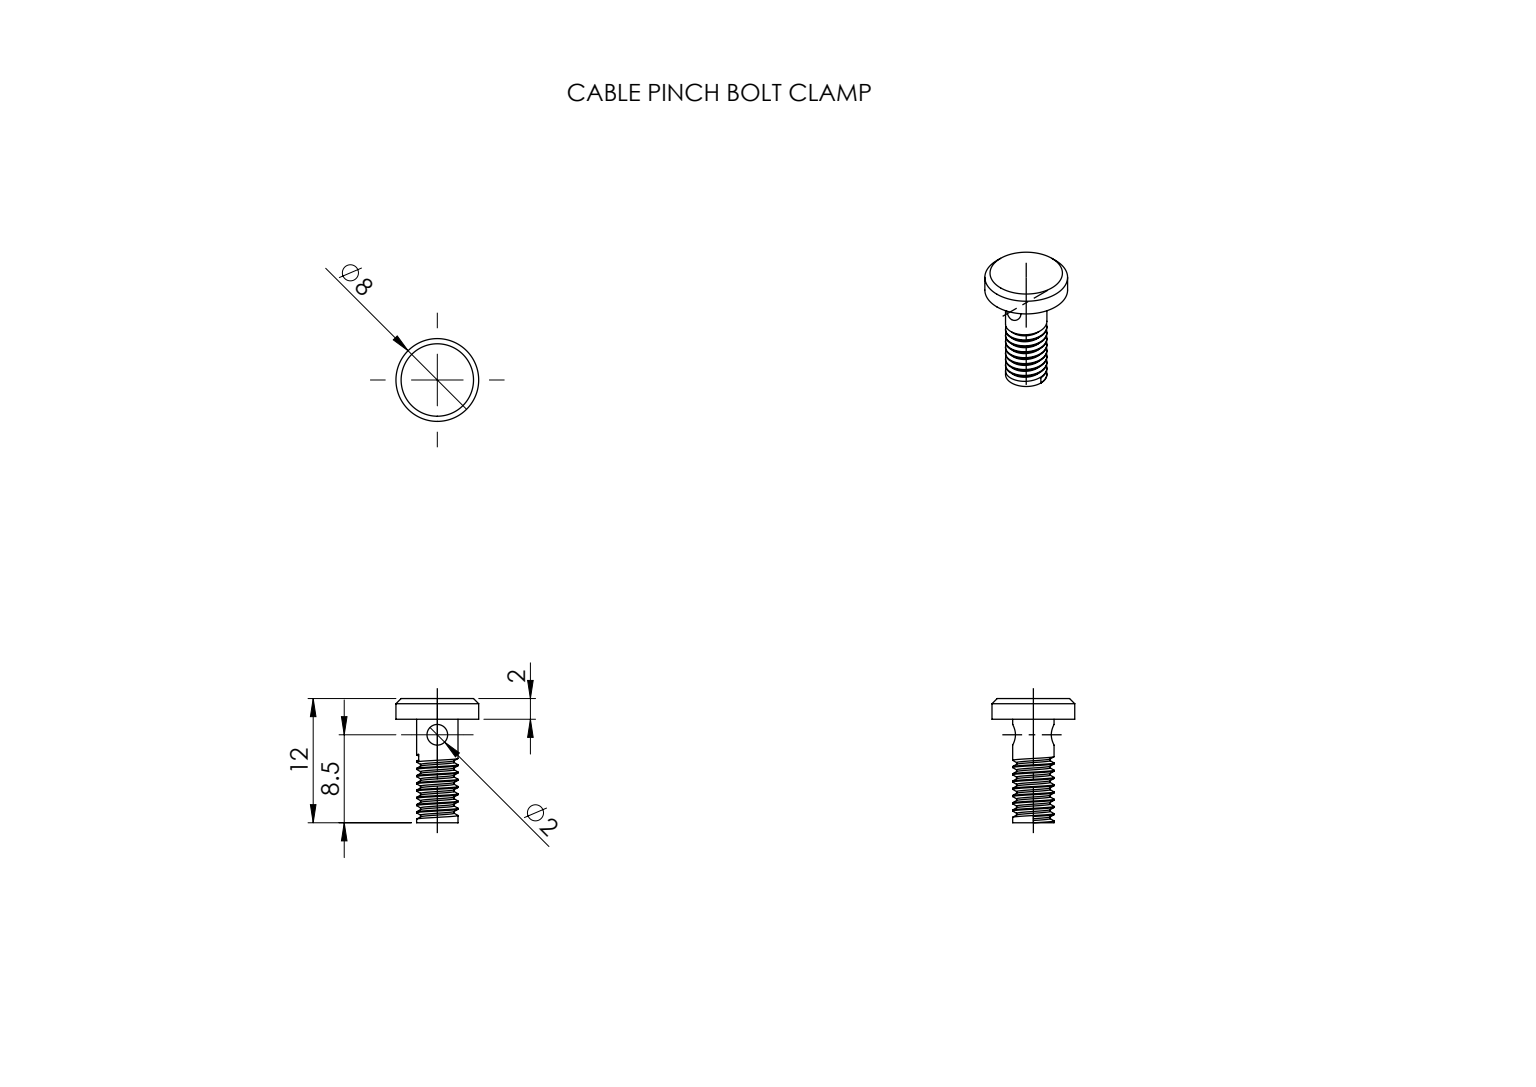
ISO-10303-21;
HEADER;
FILE_DESCRIPTION (('STEP AP214'),
    '1' );
FILE_NAME ('Cable Pinch Bolt Clamp.step',
    '2026-10-08T05:45:04',
    ( '' ),
    ( '' ),
    'SwSTEP 2.0',
    'SolidWorks 2026',
    '' );
FILE_SCHEMA (( 'AUTOMOTIVE_DESIGN' ));
ENDSEC;

DATA;
#6=CARTESIAN_POINT ( 'NONE',  ( -25.98076211353311393, 52.34374999904395054, -3.128098921329806714 ) ) ;
#9=( BOUNDED_CURVE ( )  B_SPLINE_CURVE ( 2, ( #10910, #4195, #7581, #6742, #4979, #7521, #70, #5149, #6620 ),
 .UNSPECIFIED., .F., .F. ) 
 B_SPLINE_CURVE_WITH_KNOTS ( ( 3, 2, 2, 2, 3 ),
 ( 0.6944444444444445308, 0.7037037037037037202, 0.7222222222222222099, 0.7407407407407406996, 0.7500000000000000000 ),
 .UNSPECIFIED. ) 
 CURVE ( )  GEOMETRIC_REPRESENTATION_ITEM ( )  RATIONAL_B_SPLINE_CURVE ( ( 0.9330127018922194093, 0.9330127018922197424, 1.000000000000000000, 0.8660254037844387076, 1.000000000000000000, 0.8660254037844387076, 1.000000000000000000, 0.9330127018922194093, 0.9330127018922194093 ) ) 
 REPRESENTATION_ITEM ( '' )  );
#14=DIRECTION ( 'NONE',  ( 0.000000000000000000, 0.000000000000000000, 1.000000000000000000 ) ) ;
#22=CARTESIAN_POINT ( 'NONE',  ( -24.35964822603314417, 53.91874999904395338, -5.000000000000103029 ) ) ;
#30=CARTESIAN_POINT ( 'NONE',  ( -25.98076211353311038, 60.99999999999985789, -0.9999999999995021760 ) ) ;
#31=CARTESIAN_POINT ( 'NONE',  ( -24.35964822603314772, 52.63541666571061484, -4.064049460664953983 ) ) ;
#32=CARTESIAN_POINT ( 'NONE',  ( -24.35964822603314772, 55.26041666571061484, -4.064049460664953983 ) ) ;
#35=CARTESIAN_POINT ( 'NONE',  ( -26.98076211353309972, 53.23333333333319217, -6.732050807568954909 ) ) ;
#47=CARTESIAN_POINT ( 'NONE',  ( -25.17020516978313083, 50.01041666571061484, -6.403925809002825709 ) ) ;
#52=CARTESIAN_POINT ( 'NONE',  ( -24.35964822603314417, 49.89374999904394770, -5.000000000000103029 ) ) ;
#54=ORIENTED_EDGE ( 'NONE', *, *, #4990, .T. ) ;
#62=CARTESIAN_POINT ( 'NONE',  ( -26.79131905728310059, 52.28541666571062052, -3.596074190997381237 ) ) ;
#65=CARTESIAN_POINT ( 'NONE',  ( -26.85195975805010704, 58.50831236826149251, -6.801198016534330648 ) ) ;
#67=ORIENTED_EDGE ( 'NONE', *, *, #8603, .T. ) ;
#68=AXIS2_PLACEMENT_3D ( 'NONE', #5659, #5549, #6578 ) ;
#70=CARTESIAN_POINT ( 'NONE',  ( -26.98076211353309972, 54.77916666475469754, -3.267949192431252037 ) ) ;
#74=DIRECTION ( 'NONE',  ( 1.000000000000000000, 0.000000000000000000, 0.000000000000000000 ) ) ;
#77=CARTESIAN_POINT ( 'NONE',  ( -25.98076211353311393, 55.49374999904395622, -6.871901078670400231 ) ) ;
#85=CARTESIAN_POINT ( 'NONE',  ( -25.98076211353311393, 54.22499999999985931, -3.000000000000132339 ) ) ;
#88=CARTESIAN_POINT ( 'NONE',  ( -24.35964822603314417, 52.69374999904394485, -5.000000000000103029 ) ) ;
#93=CARTESIAN_POINT ( 'NONE',  ( -27.98076211353308551, 54.69166666666652787, -6.154700538379338504 ) ) ;
#101=VERTEX_POINT ( 'NONE', #7634 ) ;
#106=CARTESIAN_POINT ( 'NONE',  ( -25.17020516978313083, 50.71041666571061057, -6.403925809002825709 ) ) ;
#111=CARTESIAN_POINT ( 'NONE',  ( -27.60187600103308014, 50.88541666571062194, -5.935950539335252074 ) ) ;
#114=CARTESIAN_POINT ( 'NONE',  ( -25.84804642293430277, 59.00000000000105871, -3.000000000000019984 ) ) ;
#123=CARTESIAN_POINT ( 'NONE',  ( -26.79131905728310059, 50.65208333237728766, -6.403925809002825709 ) ) ;
#128=ORIENTED_EDGE ( 'NONE', *, *, #2197, .F. ) ;
#130=ORIENTED_EDGE ( 'NONE', *, *, #7314, .T. ) ;
#133=DIRECTION ( 'NONE',  ( 0.000000000000000000, 1.000000000000000000, 0.000000000000000000 ) ) ;
#137=CARTESIAN_POINT ( 'NONE',  ( -26.98076211353309972, 52.76666666666653072, -3.267949192431252037 ) ) ;
#139=CARTESIAN_POINT ( 'NONE',  ( -24.35964822603314772, 54.56041666571061910, -4.064049460664953983 ) ) ;
#149=CARTESIAN_POINT ( 'NONE',  ( -24.35964822603314417, 55.49374999904394912, -5.000000000000103029 ) ) ;
#154=CARTESIAN_POINT ( 'NONE',  ( -23.98076211353314235, 54.39999999999986358, -5.000000000000103029 ) ) ;
#160=PRODUCT_CONTEXT ( 'NONE', #1750, 'mechanical' ) ;
#163=CARTESIAN_POINT ( 'NONE',  ( -23.98076211353314235, 54.34166666666652645, -3.845299461620867554 ) ) ;
#168=CARTESIAN_POINT ( 'NONE',  ( -26.79131905728310059, 53.86041666571061626, -3.596074190997381237 ) ) ;
#178=DIRECTION ( 'NONE',  ( -2.775557561562891351E-17, -1.000000000000000000, 8.326672684688671588E-17 ) ) ;
#179=CARTESIAN_POINT ( 'NONE',  ( -26.79131905728310059, 52.05208333237728624, -6.403925809002825709 ) ) ;
#186=CARTESIAN_POINT ( 'NONE',  ( -25.98076211353311393, 49.49999999999986500, -5.000000000000103029 ) ) ;
#187=FACE_OUTER_BOUND ( 'NONE', #10441, .T. ) ;
#189=CARTESIAN_POINT ( 'NONE',  ( -25.17020516978313083, 55.43541666571061910, -6.403925809002825709 ) ) ;
#190=CYLINDRICAL_SURFACE ( 'NONE', #9308, 1.999999999999971356 ) ;
#199=CARTESIAN_POINT ( 'NONE',  ( -26.98076211353408382, 57.99999999999985789, -6.732050807568389139 ) ) ;
#200=CARTESIAN_POINT ( 'NONE',  ( -23.98076211353314235, 55.15833333333319644, -6.154700538379337615 ) ) ;
#214=CARTESIAN_POINT ( 'NONE',  ( -25.98076211353311393, 54.26874999904394059, -6.871901078670400231 ) ) ;
#215=LINE ( 'NONE', #1106, #6427 ) ;
#229=CARTESIAN_POINT ( 'NONE',  ( -26.79131905728310059, 51.58541666571061768, -3.596074190997381237 ) ) ;
#232=FACE_OUTER_BOUND ( 'NONE', #6046, .T. ) ;
#239=CARTESIAN_POINT ( 'NONE',  ( -27.44132740410865523, 55.89336612041927310, -4.296608737464627126 ) ) ;
#243=SURFACE_SIDE_STYLE ('',( #1130 ) ) ;
#251=CARTESIAN_POINT ( 'NONE',  ( -26.98076211353408382, 57.86742347890963600, -6.732050807568390027 ) ) ;
#256=CARTESIAN_POINT ( 'NONE',  ( -26.98076211353309972, 55.33333333333320070, -6.732050807568954909 ) ) ;
#260=CIRCLE ( 'NONE', #5589, 4.000000000000600409 ) ;
#261=EDGE_LOOP ( 'NONE', ( #3712, #6126, #2093, #9383 ) ) ;
#273=CARTESIAN_POINT ( 'NONE',  ( -24.35964822603314772, 51.23541666571061626, -4.064049460664953983 ) ) ;
#276=VERTEX_POINT ( 'NONE', #6124 ) ;
#287=CARTESIAN_POINT ( 'NONE',  ( -27.60187600103308370, 55.66874999904394627, -5.000000000000103029 ) ) ;
#288=FACE_OUTER_BOUND ( 'NONE', #1831, .T. ) ;
#293=EDGE_CURVE ( 'NONE', #9873, #5764, #10428, .T. ) ;
#294=CARTESIAN_POINT ( 'NONE',  ( -27.78268512908116961, 55.49961679590672503, -4.132201955500060642 ) ) ;
#297=LINE ( 'NONE', #1976, #5079 ) ;
#308=AXIS2_PLACEMENT_3D ( 'NONE', #6956, #4296, #9565 ) ;
#311=CARTESIAN_POINT ( 'NONE',  ( -24.98076211353313170, 54.89583333142136468, -3.267949192431250705 ) ) ;
#313=CARTESIAN_POINT ( 'NONE',  ( -25.98076211353311393, 54.26874999904394059, -6.871901078670400231 ) ) ;
#315=AXIS2_PLACEMENT_3D ( 'NONE', #3172, #7503, #4003 ) ;
#325=CARTESIAN_POINT ( 'NONE',  ( -25.98076211353310683, 49.89374999904395480, -6.871901078670399343 ) ) ;
#328=ORIENTED_EDGE ( 'NONE', *, *, #9673, .F. ) ;
#329=CARTESIAN_POINT ( 'NONE',  ( -27.60187600103308370, 53.04374999904394627, -5.000000000000103029 ) ) ;
#339=CARTESIAN_POINT ( 'NONE',  ( -25.98076211353311393, 54.44374999904394485, -3.128098921329806714 ) ) ;
#341=CARTESIAN_POINT ( 'NONE',  ( -25.44486372867087454, 53.05623925897106830, -7.000000000000073719 ) ) ;
#357=CARTESIAN_POINT ( 'NONE',  ( -26.85338401696505883, 57.49468158336109269, -6.800474515642543238 ) ) ;
#362=CARTESIAN_POINT ( 'NONE',  ( -26.79131905728310059, 52.92708333237727913, -6.403925809002825709 ) ) ;
#367=CARTESIAN_POINT ( 'NONE',  ( -25.98076211353310683, 54.92499999999986926, -3.000000000000132339 ) ) ;
#378=CARTESIAN_POINT ( 'NONE',  ( -24.35964822603314772, 54.73541666571060915, -4.064049460664953983 ) ) ;
#388=CARTESIAN_POINT ( 'NONE',  ( -27.98076211353308551, 49.84999999999986642, -5.000000000000103029 ) ) ;
#399=CARTESIAN_POINT ( 'NONE',  ( -25.98076211353311393, 55.88749999808803182, -7.000000000000072831 ) ) ;
#404=ORIENTED_EDGE ( 'NONE', *, *, #1797, .F. ) ;
#409=EDGE_CURVE ( 'NONE', #4738, #10440, #8087, .T. ) ;
#413=CARTESIAN_POINT ( 'NONE',  ( -24.35964822603314417, 52.69374999904394485, -5.000000000000103029 ) ) ;
#433=VERTEX_POINT ( 'NONE', #9014 ) ;
#453=CARTESIAN_POINT ( 'NONE',  ( -25.44486372867087454, 52.44373926088289295, -7.000000000000073719 ) ) ;
#455=CARTESIAN_POINT ( 'NONE',  ( -25.47388223254686324, 57.12817616725342162, -6.938581062208108108 ) ) ;
#467=CARTESIAN_POINT ( 'NONE',  ( -25.44486372867087809, 52.35623925897106545, -7.000000000000075495 ) ) ;
#469=CARTESIAN_POINT ( 'NONE',  ( -23.98076211353314235, 51.54166666666652219, -3.845299461620867554 ) ) ;
#470=CARTESIAN_POINT ( 'NONE',  ( -24.35964822603314417, 53.39374999904394770, -5.000000000000103029 ) ) ;
#474=ORIENTED_EDGE ( 'NONE', *, *, #7144, .T. ) ;
#482=CARTESIAN_POINT ( 'NONE',  ( -25.98076211353310683, 51.29374999904394627, -6.871901078670399343 ) ) ;
#483=AXIS2_PLACEMENT_3D ( 'NONE', #5841, #2237, #5628 ) ;
#491=VERTEX_POINT ( 'NONE', #504 ) ;
#503=CARTESIAN_POINT ( 'NONE',  ( -27.98076211353308551, 51.80416666475470322, -6.154700538379338504 ) ) ;
#504=CARTESIAN_POINT ( 'NONE',  ( -25.98076211353311393, 51.77499999999986358, -7.000000000000072831 ) ) ;
#507=EDGE_LOOP ( 'NONE', ( #5439, #6866, #1397, #7624 ) ) ;
#509=LINE ( 'NONE', #4853, #3476 ) ;
#511=CARTESIAN_POINT ( 'NONE',  ( -27.98076211353308551, 52.50416666475469896, -6.154700538379338504 ) ) ;
#522=CARTESIAN_POINT ( 'NONE',  ( -25.98076211353311393, 51.07499999999986784, -7.000000000000073719 ) ) ;
#523=CARTESIAN_POINT ( 'NONE',  ( -24.35964822603314772, 54.03541666571061342, -4.064049460664953983 ) ) ;
#525=CARTESIAN_POINT ( 'NONE',  ( -25.98076211353311393, 49.49999999999986500, -3.000000000000131894 ) ) ;
#527=EDGE_LOOP ( 'NONE', ( #10460, #8210, #7795, #10548 ) ) ;
#533=CARTESIAN_POINT ( 'NONE',  ( -25.17020516978313083, 51.70208333237728482, -3.596074190997380349 ) ) ;
#536=CARTESIAN_POINT ( 'NONE',  ( -26.51666049839535688, 53.81876073720500386, -7.000000000000071942 ) ) ;
#543=( BOUNDED_CURVE ( )  B_SPLINE_CURVE ( 2, ( #6474, #4774, #10656, #2205, #3047, #6421, #9819, #9874, #2732 ),
 .UNSPECIFIED., .F., .F. ) 
 B_SPLINE_CURVE_WITH_KNOTS ( ( 3, 2, 2, 2, 3 ),
 ( 0.6388888888888889506, 0.6481481481481481399, 0.6666666666666666297, 0.6851851851851852304, 0.6944444444444445308 ),
 .UNSPECIFIED. ) 
 CURVE ( )  GEOMETRIC_REPRESENTATION_ITEM ( )  RATIONAL_B_SPLINE_CURVE ( ( 0.9330127018922194093, 0.9330127018922197424, 1.000000000000000000, 0.8660254037844387076, 1.000000000000000000, 0.8660254037844387076, 1.000000000000000000, 0.9330127018922189652, 0.9330127018922194093 ) ) 
 REPRESENTATION_ITEM ( '' )  );
#548=CARTESIAN_POINT ( 'NONE',  ( -23.98076211353314235, 50.81249999808803608, -5.000000000000103029 ) ) ;
#550=CARTESIAN_POINT ( 'NONE',  ( -27.44132332507749794, 55.71836679508493262, -4.296600267573891685 ) ) ;
#553=EDGE_CURVE ( 'NONE', #10440, #6171, #9641, .T. ) ;
#569=DIRECTION ( 'NONE',  ( 0.000000000000000000, 1.000000000000000000, 0.000000000000000000 ) ) ;
#574=CARTESIAN_POINT ( 'NONE',  ( -24.35964822603314417, 51.81874999904395196, -5.000000000000103029 ) ) ;
#583=CARTESIAN_POINT ( 'NONE',  ( -27.60187600103308725, 50.18541666571061199, -5.935950539335252074 ) ) ;
#584=CARTESIAN_POINT ( 'NONE',  ( -27.60187600103308370, 54.26874999904394770, -5.000000000000103029 ) ) ;
#586=CARTESIAN_POINT ( 'NONE',  ( -26.98076211353309972, 49.96666666666652645, -3.267949192431252037 ) ) ;
#587=ORIENTED_EDGE ( 'NONE', *, *, #9063, .T. ) ;
#604=CARTESIAN_POINT ( 'NONE',  ( -25.98076211353311393, 52.03749999808803040, -2.690598923241634743 ) ) ;
#612=ORIENTED_EDGE ( 'NONE', *, *, #2110, .F. ) ;
#615=CARTESIAN_POINT ( 'NONE',  ( -25.44486372867087454, 52.15626073911682425, -3.000000000000131450 ) ) ;
#634=CARTESIAN_POINT ( 'NONE',  ( -24.35964822603314772, 50.36041666571061626, -4.064049460664953983 ) ) ;
#642=CARTESIAN_POINT ( 'NONE',  ( -24.35964822603314772, 49.95208333237727771, -5.935950539335252074 ) ) ;
#643=CARTESIAN_POINT ( 'NONE',  ( -27.60187600103308725, 51.52708333237728766, -4.064049460664955760 ) ) ;
#646=CARTESIAN_POINT ( 'NONE',  ( -27.60187600103308370, 54.96874999904395054, -5.000000000000103029 ) ) ;
#648=CARTESIAN_POINT ( 'NONE',  ( -27.60187600103308370, 55.14374999904394059, -5.000000000000103029 ) ) ;
#651=DIRECTION ( 'NONE',  ( 0.000000000000000000, 0.000000000000000000, -1.000000000000000000 ) ) ;
#656=AXIS2_PLACEMENT_3D ( 'NONE', #1363, #6196, #4761 ) ;
#662=CARTESIAN_POINT ( 'NONE',  ( -24.98076211353313170, 50.69583333142136183, -3.267949192431250705 ) ) ;
#682=CARTESIAN_POINT ( 'NONE',  ( -26.51666049839536043, 52.09373926088289863, -3.000000000000133671 ) ) ;
#687=CARTESIAN_POINT ( 'NONE',  ( -24.35964822603314772, 54.73541666571060915, -4.064049460664953983 ) ) ;
#694=CARTESIAN_POINT ( 'NONE',  ( -25.98076211353310683, 51.46874999904394343, -6.871901078670399343 ) ) ;
#695=CARTESIAN_POINT ( 'NONE',  ( -26.79131905728310059, 53.68541666571061910, -3.596074190997381237 ) ) ;
#697=CARTESIAN_POINT ( 'NONE',  ( -25.98076211353311393, 52.47499999999985931, -7.309401076758571314 ) ) ;
#700=ORIENTED_EDGE ( 'NONE', *, *, #8785, .F. ) ;
#703=EDGE_CURVE ( 'NONE', #3324, #4732, #543, .T. ) ;
#711=CARTESIAN_POINT ( 'NONE',  ( -25.98076211353311393, 53.78749999808803750, -7.309401076758571314 ) ) ;
#721=VECTOR ( 'NONE', #4124, 1000.000000000000000 ) ;
#724=LINE ( 'NONE', #7457, #721 ) ;
#735=CARTESIAN_POINT ( 'NONE',  ( -25.98076211353311393, 55.88749999808803182, -7.000000000000072831 ) ) ;
#736=CARTESIAN_POINT ( 'NONE',  ( -25.98076211353311393, 50.24374999904395622, -3.128098921329806714 ) ) ;
#739=ORIENTED_EDGE ( 'NONE', *, *, #9306, .T. ) ;
#745=CARTESIAN_POINT ( 'NONE',  ( -24.35964822603314772, 54.56041666571061910, -4.064049460664953983 ) ) ;
#747=CARTESIAN_POINT ( 'NONE',  ( -23.98076211353314235, 52.29999999999986215, -5.000000000000103029 ) ) ;
#754=EDGE_CURVE ( 'NONE', #3324, #10078, #215, .T. ) ;
#764=CARTESIAN_POINT ( 'NONE',  ( -27.98076211353308551, 56.00416666475471317, -6.154700538379338504 ) ) ;
#767=DIRECTION ( 'NONE',  ( 0.000000000000000000, 1.000000000000000000, 0.000000000000000000 ) ) ;
#770=ORIENTED_EDGE ( 'NONE', *, *, #8581, .F. ) ;
#782=CARTESIAN_POINT ( 'NONE',  ( -27.98076211353308551, 55.30416666475468901, -6.154700538379338504 ) ) ;
#784=ORIENTED_EDGE ( 'NONE', *, *, #10155, .T. ) ;
#792=CARTESIAN_POINT ( 'NONE',  ( -25.44486372867087098, 55.85623925897107256, -7.000000000000071942 ) ) ;
#795=CARTESIAN_POINT ( 'NONE',  ( -27.60187600103308370, 52.86874999904394912, -5.000000000000103029 ) ) ;
#799=ORIENTED_EDGE ( 'NONE', *, *, #6532, .T. ) ;
#800=CYLINDRICAL_SURFACE ( 'NONE', #6625, 4.000000000000599520 ) ;
#801=CARTESIAN_POINT ( 'NONE',  ( -27.98076211353308551, 53.26249999808803182, -5.000000000000103029 ) ) ;
#802=CARTESIAN_POINT ( 'NONE',  ( -25.98076211353310683, 54.96874999904394343, -6.871901078670399343 ) ) ;
#808=CARTESIAN_POINT ( 'NONE',  ( -27.98076211353308551, 52.70833333333320070, -3.845299461620869330 ) ) ;
#819=CARTESIAN_POINT ( 'NONE',  ( -25.98076211353311038, 61.49999999999985789, -1.499999999999510392 ) ) ;
#822=CARTESIAN_POINT ( 'NONE',  ( -25.98076211353311393, 50.41874999904393917, -3.128098921329806714 ) ) ;
#825=B_SPLINE_CURVE_WITH_KNOTS ( 'NONE', 1,
 ( #3798, #9631 ),
 .UNSPECIFIED., .F., .F.,
 ( 2, 2 ),
 ( 0.000000000000000000, 1.000000000000000000 ),
 .UNSPECIFIED. ) ;
#827=CARTESIAN_POINT ( 'NONE',  ( -26.98076211353309972, 55.47916666475470038, -3.267949192431252037 ) ) ;
#844=CARTESIAN_POINT ( 'NONE',  ( -27.60187600103308014, 50.01041666571062194, -5.935950539335252074 ) ) ;
#859=CARTESIAN_POINT ( 'NONE',  ( -24.35964822603314772, 52.46041666571062478, -4.064049460664953983 ) ) ;
#866=CARTESIAN_POINT ( 'NONE',  ( -24.35964822603314772, 54.73541666571061626, -4.064049460664953983 ) ) ;
#868=CARTESIAN_POINT ( 'NONE',  ( -24.35964822603314772, 55.37708333237728908, -5.935950539335252074 ) ) ;
#870=CARTESIAN_POINT ( 'NONE',  ( -27.98076211353308551, 51.24999999999986500, -5.000000000000103029 ) ) ;
#871=ORIENTED_EDGE ( 'NONE', *, *, #9335, .F. ) ;
#880=CARTESIAN_POINT ( 'NONE',  ( -25.98076211353311393, 52.03749999808803750, -3.000000000000132339 ) ) ;
#881=CARTESIAN_POINT ( 'NONE',  ( -24.35964822603314417, 49.89374999904394770, -5.000000000000103029 ) ) ;
#885=CARTESIAN_POINT ( 'NONE',  ( -27.98076211353308551, 55.42083333142137036, -3.845299461620869330 ) ) ;
#888=CARTESIAN_POINT ( 'NONE',  ( -24.98076211353203746, 58.13304142775955086, -3.267949192431878203 ) ) ;
#897=CARTESIAN_POINT ( 'NONE',  ( -26.79131905728310059, 52.75208333237728198, -6.403925809002825709 ) ) ;
#902=ADVANCED_FACE ( 'NONE', ( #7791 ), #8557, .F. ) ;
#904=ORIENTED_EDGE ( 'NONE', *, *, #6155, .T. ) ;
#911=CARTESIAN_POINT ( 'NONE',  ( -27.60187600103308370, 54.96874999904395054, -5.000000000000103029 ) ) ;
#912=DIRECTION ( 'NONE',  ( 0.000000000000000000, 1.000000000000000000, 0.000000000000000000 ) ) ;
#914=LINE ( 'NONE', #2871, #8975 ) ;
#921=CARTESIAN_POINT ( 'NONE',  ( -27.60187600103308725, 52.98541666571060915, -5.935950539335252074 ) ) ;
#925=CARTESIAN_POINT ( 'NONE',  ( -26.98076211353309972, 50.66666666666652930, -3.267949192431252037 ) ) ;
#941=CARTESIAN_POINT ( 'NONE',  ( -26.98076211353309972, 55.24583333142137320, -6.732050807568954909 ) ) ;
#943=ORIENTED_EDGE ( 'NONE', *, *, #703, .F. ) ;
#944=CARTESIAN_POINT ( 'NONE',  ( -25.10950799871860184, 58.50805689774887952, -3.198836335995408398 ) ) ;
#945=ORIENTED_EDGE ( 'NONE', *, *, #2787, .F. ) ;
#952=CARTESIAN_POINT ( 'NONE',  ( -24.35964822603314772, 50.47708333237728340, -5.935950539335252074 ) ) ;
#957=ORIENTED_EDGE ( 'NONE', *, *, #2762, .T. ) ;
#958=EDGE_LOOP ( 'NONE', ( #2750, #5131, #9096, #1734 ) ) ;
#964=CARTESIAN_POINT ( 'NONE',  ( -26.98076211353309972, 52.53333333333319644, -6.732050807568954909 ) ) ;
#966=CARTESIAN_POINT ( 'NONE',  ( -26.79131905728310059, 54.15208333237728056, -6.403925809002825709 ) ) ;
#978=CARTESIAN_POINT ( 'NONE',  ( -24.35964822603314772, 55.43541666571061199, -4.064049460664953983 ) ) ;
#980=CARTESIAN_POINT ( 'NONE',  ( -23.98076211353314235, 50.95833333333318649, -6.154700538379337615 ) ) ;
#996=CARTESIAN_POINT ( 'NONE',  ( -27.60187600103308014, 51.00208333237728198, -4.064049460664955760 ) ) ;
#998=VERTEX_POINT ( 'NONE', #2847 ) ;
#1008=CARTESIAN_POINT ( 'NONE',  ( -25.98076211353311393, 51.99374999904394912, -6.871901078670400231 ) ) ;
#1022=DIRECTION ( 'NONE',  ( -0.4338606044657101757, -7.385312362483753893E-05, -0.9009800055708032662 ) ) ;
#1023=CARTESIAN_POINT ( 'NONE',  ( -24.35964822603314772, 53.97708333237728340, -5.935950539335252074 ) ) ;
#1024=LINE ( 'NONE', #7035, #2642 ) ;
#1026=DIRECTION ( 'NONE',  ( 0.000000000000000000, 1.000000000000000000, 0.000000000000000000 ) ) ;
#1033=CARTESIAN_POINT ( 'NONE',  ( -25.17020516978313083, 55.37708333237728198, -3.596074190997380349 ) ) ;
#1034=CARTESIAN_POINT ( 'NONE',  ( -24.98076211353313170, 54.98333333333319928, -3.267949192431250705 ) ) ;
#1041=CARTESIAN_POINT ( 'NONE',  ( -27.98076211353308551, 54.69166666666652787, -6.154700538379338504 ) ) ;
#1042=EDGE_CURVE ( 'NONE', #5004, #1390, #1912, .T. ) ;
#1047=CARTESIAN_POINT ( 'NONE',  ( -25.44486372867087809, 54.25626073911683278, -3.000000000000132339 ) ) ;
#1050=CARTESIAN_POINT ( 'NONE',  ( -24.35964822603314772, 53.33541666571061057, -4.064049460664953983 ) ) ;
#1062=CARTESIAN_POINT ( 'NONE',  ( -27.60187600103308014, 51.41041666571062052, -5.935950539335252074 ) ) ;
#1073=CARTESIAN_POINT ( 'NONE',  ( -26.98076211353408738, 58.13236904469467703, -3.267949192431818695 ) ) ;
#1086=CARTESIAN_POINT ( 'NONE',  ( -25.44486372867087809, 53.75623925897105693, -7.000000000000075495 ) ) ;
#1088=CARTESIAN_POINT ( 'NONE',  ( -25.98076211353311038, 59.49999999999985789, -0.9999999999995021760 ) ) ;
#1089=CARTESIAN_POINT ( 'NONE',  ( -24.98076211353313170, 54.28333333333319644, -3.267949192431250705 ) ) ;
#1099=CARTESIAN_POINT ( 'NONE',  ( -26.51666049839535688, 51.71876073720500955, -7.000000000000074607 ) ) ;
#1105=CARTESIAN_POINT ( 'NONE',  ( -24.35964822603314772, 52.63541666571061484, -4.064049460664953983 ) ) ;
#1106=CARTESIAN_POINT ( 'NONE',  ( -25.98076211353311393, 49.49999999999986500, -3.000000000000131894 ) ) ;
#1119=CARTESIAN_POINT ( 'NONE',  ( -25.98076211353311393, 53.74374999904394912, -3.128098921329806714 ) ) ;
#1121=CARTESIAN_POINT ( 'NONE',  ( -25.44486372867087454, 50.25623925897107114, -7.000000000000073719 ) ) ;
#1122=DIRECTION ( 'NONE',  ( 0.000000000000000000, 0.000000000000000000, 1.000000000000000000 ) ) ;
#1129=CARTESIAN_POINT ( 'NONE',  ( -27.44132332507749439, 55.71836679508493972, -4.296600267573891685 ) ) ;
#1130=SURFACE_STYLE_FILL_AREA ( #1928 ) ;
#1142=CARTESIAN_POINT ( 'NONE',  ( -26.79131905728310059, 53.86041666571061626, -3.596074190997381237 ) ) ;
#1144=CARTESIAN_POINT ( 'NONE',  ( -27.98076211353308551, 54.74999999999985789, -5.000000000000103029 ) ) ;
#1148=( BOUNDED_CURVE ( )  B_SPLINE_CURVE ( 2, ( #2992, #10744, #9970, #3087, #7467, #6517, #1527, #467, #1368 ),
 .UNSPECIFIED., .F., .F. ) 
 B_SPLINE_CURVE_WITH_KNOTS ( ( 3, 2, 2, 2, 3 ),
 ( 0.3055555555555555802, 0.3148148148148148251, 0.3333333333333333148, 0.3518518518518518601, 0.3611111111111111605 ),
 .UNSPECIFIED. ) 
 CURVE ( )  GEOMETRIC_REPRESENTATION_ITEM ( )  RATIONAL_B_SPLINE_CURVE ( ( 0.9330127018922194093, 0.9330127018922195203, 1.000000000000000000, 0.8660254037844387076, 1.000000000000000000, 0.8660254037844387076, 1.000000000000000000, 0.9330127018922189652, 0.9330127018922194093 ) ) 
 REPRESENTATION_ITEM ( '' )  );
#1161=CARTESIAN_POINT ( 'NONE',  ( -24.35964822603314772, 51.35208333237728340, -5.935950539335252074 ) ) ;
#1174=CARTESIAN_POINT ( 'NONE',  ( -26.79131905728310059, 55.08541666571061768, -3.596074190997381237 ) ) ;
#1181=EDGE_CURVE ( 'NONE', #3014, #7830, #1772, .T. ) ;
#1183=CARTESIAN_POINT ( 'NONE',  ( -25.98076211353311393, 49.49999999999986500, -3.000000000000131894 ) ) ;
#1184=CARTESIAN_POINT ( 'NONE',  ( -24.98076211353313170, 50.08333333333319359, -3.267949192431250705 ) ) ;
#1188=LINE ( 'NONE', #1248, #10504 ) ;
#1192=ORIENTED_EDGE ( 'NONE', *, *, #2878, .T. ) ;
#1200=CARTESIAN_POINT ( 'NONE',  ( -27.60187600103308370, 55.86681146796336606, -4.629981812462977686 ) ) ;
#1204=CARTESIAN_POINT ( 'NONE',  ( -25.98076211353311393, 52.16874999904393917, -6.871901078670400231 ) ) ;
#1208=COLOUR_RGB ( '', 0.66274510, 0.83137255, 0.94901961) ;
#1212=ORIENTED_EDGE ( 'NONE', *, *, #2230, .F. ) ;
#1213=CARTESIAN_POINT ( 'NONE',  ( -23.98076211353314235, 50.87083333142136610, -6.154700538379337615 ) ) ;
#1214=DIRECTION ( 'NONE',  ( 0.000000000000000000, 0.000000000000000000, -1.000000000000000000 ) ) ;
#1218=CARTESIAN_POINT ( 'NONE',  ( -25.98076211353311393, 52.03749999808803750, -3.000000000000132783 ) ) ;
#1225=CARTESIAN_POINT ( 'NONE',  ( -27.60187600103308014, 53.80208333237727203, -4.064049460664955760 ) ) ;
#1235=CARTESIAN_POINT ( 'NONE',  ( -25.98076211353311393, 53.39374999904394770, -6.871901078670400231 ) ) ;
#1239=CARTESIAN_POINT ( 'NONE',  ( -25.98076211353311393, 59.00000000000083134, -7.000000000000074607 ) ) ;
#1241=ORIENTED_EDGE ( 'NONE', *, *, #6072, .T. ) ;
#1248=CARTESIAN_POINT ( 'NONE',  ( -23.98076211353314235, 49.49999999999986500, -5.000000000000103029 ) ) ;
#1251=CARTESIAN_POINT ( 'NONE',  ( -24.98076211353312814, 49.61666666666653214, -6.732050807568954909 ) ) ;
#1260=CARTESIAN_POINT ( 'NONE',  ( -26.11400170334226445, 56.99999999999887734, -7.000000000000075495 ) ) ;
#1261=CARTESIAN_POINT ( 'NONE',  ( -25.98076211353311393, 53.17499999999985505, -7.000000000000072831 ) ) ;
#1264=CARTESIAN_POINT ( 'NONE',  ( -27.60187600103308014, 52.40208333237728056, -4.064049460664955760 ) ) ;
#1287=( NAMED_UNIT ( * ) PLANE_ANGLE_UNIT ( ) SI_UNIT ( $, .RADIAN. ) );
#1302=CARTESIAN_POINT ( 'NONE',  ( -25.10912755541051666, 57.49274335135479674, -6.800970407759691305 ) ) ;
#1306=ORIENTED_EDGE ( 'NONE', *, *, #6540, .T. ) ;
#1310=CARTESIAN_POINT ( 'NONE',  ( -25.98076211353311393, 50.72499999999985931, -3.000000000000132783 ) ) ;
#1311=CARTESIAN_POINT ( 'NONE',  ( -23.98076211353314235, 53.67083333142137036, -6.154700538379337615 ) ) ;
#1312=CARTESIAN_POINT ( 'NONE',  ( -25.44486372867087098, 51.45626073911682852, -3.000000000000133227 ) ) ;
#1313=CARTESIAN_POINT ( 'NONE',  ( -24.35964822603314417, 51.29374999904394627, -5.000000000000103029 ) ) ;
#1326=CARTESIAN_POINT ( 'NONE',  ( -24.35964822603314417, 49.71874999904395054, -5.000000000000103029 ) ) ;
#1340=PRESENTATION_STYLE_ASSIGNMENT (( #8848 ) ) ;
#1346=AXIS2_PLACEMENT_3D ( 'NONE', #6919, #7587, #74 ) ;
#1347=CARTESIAN_POINT ( 'NONE',  ( -25.98076211353311393, 50.98749999808803324, -7.309401076758571314 ) ) ;
#1350=CARTESIAN_POINT ( 'NONE',  ( -25.98076211353311393, 52.73749999808803324, -3.000000000000132339 ) ) ;
#1357=CARTESIAN_POINT ( 'NONE',  ( -26.51666049839535688, 49.99373926088290432, -3.000000000000134115 ) ) ;
#1358=CARTESIAN_POINT ( 'NONE',  ( -25.71440107481355142, 57.02734599875091703, -6.985969673875411345 ) ) ;
#1363=CARTESIAN_POINT ( 'NONE',  ( -25.98076211353311038, 60.99999999999985789, -5.000000000000102141 ) ) ;
#1364=AXIS2_PLACEMENT_3D ( 'NONE', #6237, #133, #6290 ) ;
#1368=CARTESIAN_POINT ( 'NONE',  ( -25.98076211353311393, 52.38749999808802471, -7.000000000000072831 ) ) ;
#1371=CARTESIAN_POINT ( 'NONE',  ( -25.17020516978313083, 53.97708333237728340, -3.596074190997380349 ) ) ;
#1379=CARTESIAN_POINT ( 'NONE',  ( -25.98076211353311393, 49.49999999999986500, -5.000000000000103029 ) ) ;
#1382=CARTESIAN_POINT ( 'NONE',  ( -24.35964822603314772, 52.05208333237727913, -5.935950539335252074 ) ) ;
#1383=CARTESIAN_POINT ( 'NONE',  ( -27.60187600103308725, 51.41041666571062052, -5.935950539335252074 ) ) ;
#1387=B_SPLINE_CURVE_WITH_KNOTS ( 'NONE', 3,
 ( #1672, #888, #4236, #944, #3458, #6839, #8452, #7735, #114, #2629 ),
 .UNSPECIFIED., .F., .F.,
 ( 4, 2, 2, 2, 4 ),
 ( 0.001591453205566317926, 0.001988835618581903577, 0.002386218031597489228, 0.002783600444613075313, 0.003180982857628660964 ),
 .UNSPECIFIED. ) ;
#1390=VERTEX_POINT ( 'NONE', #1088 ) ;
#1397=ORIENTED_EDGE ( 'NONE', *, *, #4683, .T. ) ;
#1398=VECTOR ( 'NONE', #912, 1000.000000000000000 ) ;
#1403=CARTESIAN_POINT ( 'NONE',  ( -27.98076211353308551, 53.26249999808803182, -5.000000000000103029 ) ) ;
#1411=CARTESIAN_POINT ( 'NONE',  ( -27.78269984933782411, 56.11211482050296695, -4.132232521764788835 ) ) ;
#1422=CARTESIAN_POINT ( 'NONE',  ( -23.98076211353314235, 49.49999999999986500, -5.000000000000103029 ) ) ;
#1425=CARTESIAN_POINT ( 'NONE',  ( -26.79131905728310059, 51.58541666571061768, -3.596074190997381237 ) ) ;
#1430=CYLINDRICAL_SURFACE ( 'NONE', #2561, 1.999999999999971356 ) ;
#1431=DIRECTION ( 'NONE',  ( -0.000000000000000000, -0.000000000000000000, 1.000000000000000000 ) ) ;
#1432=CARTESIAN_POINT ( 'NONE',  ( -26.79131905728310059, 55.08541666571061768, -3.596074190997381237 ) ) ;
#1435=CARTESIAN_POINT ( 'NONE',  ( -27.60187600103308014, 54.32708333237728482, -4.064049460664955760 ) ) ;
#1451=CARTESIAN_POINT ( 'NONE',  ( -23.98076211353314235, 51.57083333142137604, -6.154700538379337615 ) ) ;
#1461=CARTESIAN_POINT ( 'NONE',  ( -24.98076211353312814, 52.41666666666652930, -6.732050807568954909 ) ) ;
#1464=CARTESIAN_POINT ( 'NONE',  ( -26.98076211353408382, 57.99999999999985789, -3.267949192431818251 ) ) ;
#1468=CARTESIAN_POINT ( 'NONE',  ( -27.98076211353308551, 55.42083333142136325, -3.845299461620869330 ) ) ;
#1475=CARTESIAN_POINT ( 'NONE',  ( -24.35964822603314417, 51.11874999904394912, -5.000000000000103029 ) ) ;
#1481=CARTESIAN_POINT ( 'NONE',  ( -27.60187600103308725, 51.00208333237728198, -4.064049460664955760 ) ) ;
#1482=CARTESIAN_POINT ( 'NONE',  ( -27.60187600103308725, 52.81041666571061199, -5.935950539335252074 ) ) ;
#1484=CARTESIAN_POINT ( 'NONE',  ( -27.60187600103308370, 54.26874999904394770, -5.000000000000103029 ) ) ;
#1486=CARTESIAN_POINT ( 'NONE',  ( -24.35964822603314772, 55.55208333237727913, -5.935950539335252074 ) ) ;
#1490=FACE_OUTER_BOUND ( 'NONE', #9004, .T. ) ;
#1492=DIRECTION ( 'NONE',  ( 0.000000000000000000, 8.326672684688671588E-17, 1.000000000000000000 ) ) ;
#1501=CARTESIAN_POINT ( 'NONE',  ( -26.98076211353309972, 51.97916666475470038, -3.267949192431252037 ) ) ;
#1504=CARTESIAN_POINT ( 'NONE',  ( -26.98076211353309972, 51.27916666475469754, -3.267949192431252037 ) ) ;
#1512=CARTESIAN_POINT ( 'NONE',  ( -25.98076211353311393, 49.49999999999986500, -7.000000000000074607 ) ) ;
#1514=DIRECTION ( 'NONE',  ( 0.000000000000000000, 0.000000000000000000, 1.000000000000000000 ) ) ;
#1527=CARTESIAN_POINT ( 'NONE',  ( -24.98076211353312814, 52.32916666475470180, -6.732050807568954909 ) ) ;
#1530=CARTESIAN_POINT ( 'NONE',  ( -27.60187600103308014, 50.82708333237729192, -4.064049460664955760 ) ) ;
#1537=EDGE_CURVE ( 'NONE', #9017, #10440, #7362, .T. ) ;
#1538=CARTESIAN_POINT ( 'NONE',  ( -25.17020516978313083, 51.17708333237727913, -3.596074190997380349 ) ) ;
#1539=CARTESIAN_POINT ( 'NONE',  ( -24.35964822603314772, 51.87708333237728198, -5.935950539335252074 ) ) ;
#1543=CARTESIAN_POINT ( 'NONE',  ( -24.98076211353313170, 52.18333333333320212, -3.267949192431250705 ) ) ;
#1546=EDGE_CURVE ( 'NONE', #998, #4861, #8541, .T. ) ;
#1558=CARTESIAN_POINT ( 'NONE',  ( -24.98076211353313170, 51.39583333142136468, -3.267949192431250705 ) ) ;
#1585=CARTESIAN_POINT ( 'NONE',  ( -24.35964822603314417, 55.49374999904394912, -5.000000000000103029 ) ) ;
#1593=CARTESIAN_POINT ( 'NONE',  ( -25.98076211353310683, 51.81874999904394485, -3.128098921329806714 ) ) ;
#1595=CARTESIAN_POINT ( 'NONE',  ( -27.60187600103308725, 54.21041666571061768, -5.935950539335252074 ) ) ;
#1597=CARTESIAN_POINT ( 'NONE',  ( -27.98076211353308551, 53.34999999999985931, -5.000000000000103029 ) ) ;
#1598=VERTEX_POINT ( 'NONE', #2361 ) ;
#1614=CARTESIAN_POINT ( 'NONE',  ( -26.98076211353309972, 54.54583333142136325, -6.732050807568954909 ) ) ;
#1627=( BOUNDED_CURVE ( )  B_SPLINE_CURVE ( 2, ( #522, #3090, #10651, #3968, #3764, #4711, #10490, #7202, #5543 ),
 .UNSPECIFIED., .F., .F. ) 
 B_SPLINE_CURVE_WITH_KNOTS ( ( 3, 2, 2, 2, 3 ),
 ( 0.2500000000000000000, 0.2592592592592592449, 0.2777777777777777901, 0.2962962962962962798, 0.3055555555555555802 ),
 .UNSPECIFIED. ) 
 CURVE ( )  GEOMETRIC_REPRESENTATION_ITEM ( )  RATIONAL_B_SPLINE_CURVE ( ( 0.9330127018922192983, 0.9330127018922194093, 1.000000000000000000, 0.8660254037844387076, 1.000000000000000000, 0.8660254037844387076, 1.000000000000000000, 0.9330127018922191873, 0.9330127018922194093 ) ) 
 REPRESENTATION_ITEM ( '' )  );
#1628=CARTESIAN_POINT ( 'NONE',  ( -24.98076211353213694, 57.99999999999985789, -6.732050807568384698 ) ) ;
#1633=CARTESIAN_POINT ( 'NONE',  ( -25.98076211353311393, 50.28749999808804461, -7.000000000000073719 ) ) ;
#1640=CARTESIAN_POINT ( 'NONE',  ( -23.98076211353314235, 55.65416666475469754, -3.845299461620867554 ) ) ;
#1642=CARTESIAN_POINT ( 'NONE',  ( -25.17020516978313083, 54.67708333237727913, -3.596074190997380349 ) ) ;
#1644=DIRECTION ( 'NONE',  ( 0.000000000000000000, 0.000000000000000000, -1.000000000000000000 ) ) ;
#1647=CARTESIAN_POINT ( 'NONE',  ( -27.98076211353308551, 50.60833333333319928, -3.845299461620869330 ) ) ;
#1649=CARTESIAN_POINT ( 'NONE',  ( -25.98076211353310683, 55.66874999904395338, -6.871901078670399343 ) ) ;
#1650=CARTESIAN_POINT ( 'NONE',  ( -24.35964822603314772, 51.76041666571061484, -4.064049460664953983 ) ) ;
#1652=CARTESIAN_POINT ( 'NONE',  ( -24.98076211353312814, 53.81666666666652787, -6.732050807568954909 ) ) ;
#1666=CARTESIAN_POINT ( 'NONE',  ( -26.79131905728310059, 50.12708333237728198, -6.403925809002825709 ) ) ;
#1669=CARTESIAN_POINT ( 'NONE',  ( -27.78269016046133544, 56.11211611946337285, -4.132212402892765368 ) ) ;
#1672=CARTESIAN_POINT ( 'NONE',  ( -24.98076211353193798, 57.99999999999910472, -3.267949192431741423 ) ) ;
#1675=ORIENTED_EDGE ( 'NONE', *, *, #4069, .F. ) ;
#1679=CARTESIAN_POINT ( 'NONE',  ( -25.98076211353311393, 51.68749999808803608, -7.000000000000073719 ) ) ;
#1680=CARTESIAN_POINT ( 'NONE',  ( -25.98076211353311393, 51.64374999904395480, -3.128098921329806714 ) ) ;
#1698=CARTESIAN_POINT ( 'NONE',  ( -26.79131905728310059, 52.75208333237728198, -6.403925809002825709 ) ) ;
#1705=DIRECTION ( 'NONE',  ( -2.775557561562891351E-17, -1.000000000000000000, 8.326672684688671588E-17 ) ) ;
#1707=CARTESIAN_POINT ( 'NONE',  ( -24.35964822603314772, 54.03541666571062052, -4.064049460664953983 ) ) ;
#1711=CARTESIAN_POINT ( 'NONE',  ( -27.98076211353308551, 54.04999999999986215, -5.000000000000103029 ) ) ;
#1722=CARTESIAN_POINT ( 'NONE',  ( -25.98076211353311393, 55.18749999808803608, -7.000000000000072831 ) ) ;
#1723=ORIENTED_EDGE ( 'NONE', *, *, #9806, .T. ) ;
#1730=CARTESIAN_POINT ( 'NONE',  ( -25.17020516978313083, 50.71041666571061057, -6.403925809002825709 ) ) ;
#1734=ORIENTED_EDGE ( 'NONE', *, *, #10284, .F. ) ;
#1738=VERTEX_POINT ( 'NONE', #4261 ) ;
#1740=EDGE_CURVE ( 'NONE', #8489, #6512, #6695, .T. ) ;
#1741=LINE ( 'NONE', #8396, #7743 ) ;
#1749=CARTESIAN_POINT ( 'NONE',  ( -26.97398308763695596, 58.13372405103771001, -6.736012309356057770 ) ) ;
#1750=APPLICATION_CONTEXT ( 'automotive_design' ) ;
#1757=CARTESIAN_POINT ( 'NONE',  ( -25.98076211353311393, 49.49999999999986500, -3.000000000000131894 ) ) ;
#1762=CARTESIAN_POINT ( 'NONE',  ( -27.60187600103308014, 54.91041666571061342, -5.935950539335252074 ) ) ;
#1770=CARTESIAN_POINT ( 'NONE',  ( -24.35964822603314417, 53.39374999904394770, -5.000000000000103029 ) ) ;
#1772=LINE ( 'NONE', #3549, #9979 ) ;
#1773=CARTESIAN_POINT ( 'NONE',  ( -27.98076211353308551, 50.60833333333320638, -3.845299461620869330 ) ) ;
#1780=ORIENTED_EDGE ( 'NONE', *, *, #8238, .F. ) ;
#1785=DIRECTION ( 'NONE',  ( -2.775557561562891351E-17, -1.000000000000000000, 8.326672684688671588E-17 ) ) ;
#1788=CARTESIAN_POINT ( 'NONE',  ( -27.98076211353308551, 53.90416666475469754, -6.154700538379338504 ) ) ;
#1796=EDGE_CURVE ( 'NONE', #8872, #5599, #7668, .T. ) ;
#1797=EDGE_CURVE ( 'NONE', #2436, #2510, #1024, .T. ) ;
#1800=FACE_OUTER_BOUND ( 'NONE', #3769, .T. ) ;
#1803=CARTESIAN_POINT ( 'NONE',  ( -26.59672572989580175, 58.79818731520758490, -6.905264038683467831 ) ) ;
#1811=FACE_OUTER_BOUND ( 'NONE', #527, .T. ) ;
#1812=CARTESIAN_POINT ( 'NONE',  ( -25.17020516978313083, 53.10208333237728340, -3.596074190997380349 ) ) ;
#1813=CARTESIAN_POINT ( 'NONE',  ( -25.98076211353311393, 49.49999999999986500, -3.000000000000131894 ) ) ;
#1820=CARTESIAN_POINT ( 'NONE',  ( -27.60187600103308725, 55.08541666571062478, -5.935950539335252074 ) ) ;
#1824=CARTESIAN_POINT ( 'NONE',  ( -25.98076211353311393, 49.49999999999986500, -5.000000000000103029 ) ) ;
#1826=ORIENTED_EDGE ( 'NONE', *, *, #8639, .T. ) ;
#1827=ORIENTED_EDGE ( 'NONE', *, *, #10610, .T. ) ;
#1831=EDGE_LOOP ( 'NONE', ( #6646, #1826, #784, #612, #9485, #3243, #4119, #8001, #943, #9944, #8294, #9926, #3834, #945, #700, #871, #8492, #2455, #6586, #5020, #1905 ) ) ;
#1838=CARTESIAN_POINT ( 'NONE',  ( -26.98076211353309972, 55.94583333142136894, -6.732050807568954909 ) ) ;
#1846=MANIFOLD_SOLID_BREP ( 'Cut-Extrude1', #8957 ) ;
#1847=CARTESIAN_POINT ( 'NONE',  ( -25.71518008040301240, 58.97299622964627730, -6.986129658743783999 ) ) ;
#1849=CARTESIAN_POINT ( 'NONE',  ( -25.98076211353311393, 50.94374999904395196, -3.128098921329806714 ) ) ;
#1858=DIRECTION ( 'NONE',  ( 0.000000000000000000, 1.000000000000000000, 0.000000000000000000 ) ) ;
#1859=VECTOR ( 'NONE', #10695, 1000.000000000000000 ) ;
#1863=CARTESIAN_POINT ( 'NONE',  ( -26.79131905728310059, 54.38541666571061484, -3.596074190997381237 ) ) ;
#1877=VECTOR ( 'NONE', #4617, 1000.000000000000000 ) ;
#1878=CARTESIAN_POINT ( 'NONE',  ( -26.79131905728310059, 53.16041666571061342, -3.596074190997381237 ) ) ;
#1879=CARTESIAN_POINT ( 'NONE',  ( -27.60187600103308370, 55.66874999904394627, -5.000000000000103029 ) ) ;
#1883=CARTESIAN_POINT ( 'NONE',  ( -27.98076211353308196, 55.47306177707831409, -4.543495204426306167 ) ) ;
#1886=ORIENTED_EDGE ( 'NONE', *, *, #10803, .T. ) ;
#1887=CYLINDRICAL_SURFACE ( 'NONE', #10365, 1.999999999999971356 ) ;
#1900=CARTESIAN_POINT ( 'NONE',  ( -26.79131905728310059, 53.16041666571061342, -3.596074190997381237 ) ) ;
#1902=ORIENTED_EDGE ( 'NONE', *, *, #2908, .T. ) ;
#1904=AXIS2_PLACEMENT_3D ( 'NONE', #7251, #569, #9127 ) ;
#1905=ORIENTED_EDGE ( 'NONE', *, *, #293, .F. ) ;
#1912=LINE ( 'NONE', #7745, #5203 ) ;
#1918=EDGE_LOOP ( 'NONE', ( #10991, #6008, #3805, #6399 ) ) ;
#1920=DIRECTION ( 'NONE',  ( 0.000000000000000000, 0.000000000000000000, 1.000000000000000000 ) ) ;
#1922=VECTOR ( 'NONE', #1785, 1000.000000000000000 ) ;
#1925=CARTESIAN_POINT ( 'NONE',  ( -26.48997544305390051, 58.87073604165634322, -3.061924168864667894 ) ) ;
#1927=CARTESIAN_POINT ( 'NONE',  ( -25.17020516978313083, 52.40208333237728766, -3.596074190997380349 ) ) ;
#1928=FILL_AREA_STYLE ('',( #2820 ) ) ;
#1935=CARTESIAN_POINT ( 'NONE',  ( -25.98076211353311393, 53.43749999808803608, -3.000000000000132339 ) ) ;
#1938=CARTESIAN_POINT ( 'NONE',  ( -25.44486372867087809, 54.86876073720499392, -3.000000000000132339 ) ) ;
#1944=VERTEX_POINT ( 'NONE', #3393 ) ;
#1945=( BOUNDED_CURVE ( )  B_SPLINE_CURVE ( 2, ( #6608, #615, #10729, #3854, #4011, #7397, #1461, #453, #6503 ),
 .UNSPECIFIED., .F., .F. ) 
 B_SPLINE_CURVE_WITH_KNOTS ( ( 3, 2, 2, 2, 3 ),
 ( 0.4166666666666666297, 0.4259259259259259300, 0.4444444444444444198, 0.4629629629629629650, 0.4722222222222222099 ),
 .UNSPECIFIED. ) 
 CURVE ( )  GEOMETRIC_REPRESENTATION_ITEM ( )  RATIONAL_B_SPLINE_CURVE ( ( 0.9330127018922194093, 0.9330127018922191873, 1.000000000000000000, 0.8660254037844387076, 1.000000000000000000, 0.8660254037844387076, 1.000000000000000000, 0.9330127018922194093, 0.9330127018922194093 ) ) 
 REPRESENTATION_ITEM ( '' )  );
#1947=CARTESIAN_POINT ( 'NONE',  ( -26.98076211353309972, 54.86666666666653214, -3.267949192431252037 ) ) ;
#1952=FACE_OUTER_BOUND ( 'NONE', #3781, .T. ) ;
#1957=CARTESIAN_POINT ( 'NONE',  ( -27.60187600103308014, 52.40208333237728056, -4.064049460664955760 ) ) ;
#1961=ORIENTED_EDGE ( 'NONE', *, *, #10826, .F. ) ;
#1965=CARTESIAN_POINT ( 'NONE',  ( -25.98076211353311393, 49.49999999999986500, -5.000000000000103029 ) ) ;
#1967=CARTESIAN_POINT ( 'NONE',  ( -25.17020516978313083, 53.33541666571061768, -6.403925809002825709 ) ) ;
#1974=CARTESIAN_POINT ( 'NONE',  ( -25.98076211353311393, 49.49999999999986500, -3.000000000000131894 ) ) ;
#1976=CARTESIAN_POINT ( 'NONE',  ( -25.98076211353311393, 49.49999999999986500, -7.000000000000074607 ) ) ;
#1988=AXIS2_PLACEMENT_3D ( 'NONE', #1824, #7049, #6206 ) ;
#1989=CARTESIAN_POINT ( 'NONE',  ( -26.79131905728310059, 51.06041666571061199, -3.596074190997381237 ) ) ;
#1991=CARTESIAN_POINT ( 'NONE',  ( -25.98076211353311393, 55.27499999999986358, -7.309401076758571314 ) ) ;
#2004=CARTESIAN_POINT ( 'NONE',  ( -24.35964822603314772, 53.45208333237727771, -5.935950539335252074 ) ) ;
#2016=CARTESIAN_POINT ( 'NONE',  ( -26.79131905728310059, 53.45208333237728482, -6.403925809002825709 ) ) ;
#2019=EDGE_LOOP ( 'NONE', ( #8209, #7298, #5855, #6764 ) ) ;
#2020=DIRECTION ( 'NONE',  ( 0.000000000000000000, 0.000000000000000000, 1.000000000000000000 ) ) ;
#2024=CARTESIAN_POINT ( 'NONE',  ( -26.98076211353309972, 55.94583333142136894, -6.732050807568954909 ) ) ;
#2025=CARTESIAN_POINT ( 'NONE',  ( -26.98076211353309972, 52.67916666475470322, -3.267949192431252037 ) ) ;
#2041=CARTESIAN_POINT ( 'NONE',  ( -25.17020516978313083, 51.87708333237728198, -3.596074190997380349 ) ) ;
#2043=CARTESIAN_POINT ( 'NONE',  ( -25.98076211353311393, 54.22499999999986642, -2.690598923241634743 ) ) ;
#2054=CARTESIAN_POINT ( 'NONE',  ( -27.60187600103308725, 50.71041666571061768, -5.935950539335252074 ) ) ;
#2059=CARTESIAN_POINT ( 'NONE',  ( -25.17020516978313083, 52.11041666571060915, -6.403925809002825709 ) ) ;
#2073=CARTESIAN_POINT ( 'NONE',  ( -27.60187600103308014, 54.91041666571061342, -5.935950539335252074 ) ) ;
#2075=CARTESIAN_POINT ( 'NONE',  ( -23.98076211353314235, 50.11249999808803324, -5.000000000000103029 ) ) ;
#2078=EDGE_LOOP ( 'NONE', ( #904, #5617, #328, #7180 ) ) ;
#2082=CARTESIAN_POINT ( 'NONE',  ( -23.98076211353314235, 50.25833333333320496, -6.154700538379337615 ) ) ;
#2084=CARTESIAN_POINT ( 'NONE',  ( -25.98076211353311393, 53.87499999999986500, -7.000000000000072831 ) ) ;
#2093=ORIENTED_EDGE ( 'NONE', *, *, #9306, .F. ) ;
#2096=AXIS2_PLACEMENT_3D ( 'NONE', #1965, #5299, #8685 ) ;
#2099=CARTESIAN_POINT ( 'NONE',  ( -27.60187600103308370, 55.84374999904394343, -5.000000000000103029 ) ) ;
#2100=CARTESIAN_POINT ( 'NONE',  ( -24.98076211353312814, 53.11666666666652503, -6.732050807568954909 ) ) ;
#2102=CARTESIAN_POINT ( 'NONE',  ( -26.79131905728310059, 51.52708333237728056, -6.403925809002825709 ) ) ;
#2110=EDGE_CURVE ( 'NONE', #2436, #9774, #4753, .T. ) ;
#2120=CARTESIAN_POINT ( 'NONE',  ( -24.35964822603314417, 51.29374999904394627, -5.000000000000103029 ) ) ;
#2121=EDGE_LOOP ( 'NONE', ( #4568, #2616, #10712, #10894 ) ) ;
#2137=CARTESIAN_POINT ( 'NONE',  ( -25.98076211353311393, 59.49999999999985789, -7.000000000000074607 ) ) ;
#2151=CARTESIAN_POINT ( 'NONE',  ( -27.44132740410865523, 55.89336612041927310, -4.296608737464627126 ) ) ;
#2152=CARTESIAN_POINT ( 'NONE',  ( -23.98076211353314235, 53.61249999808804034, -5.000000000000103029 ) ) ;
#2153=CARTESIAN_POINT ( 'NONE',  ( -26.79131905728310059, 53.16041666571061342, -3.596074190997381237 ) ) ;
#2163=CARTESIAN_POINT ( 'NONE',  ( -26.79131905728310059, 50.18541666571061199, -3.596074190997381237 ) ) ;
#2177=CARTESIAN_POINT ( 'NONE',  ( -27.98076211353308551, 52.56249999808803608, -5.000000000000103029 ) ) ;
#2180=CARTESIAN_POINT ( 'NONE',  ( -26.11323168687438212, 59.00000000000083134, -7.000000000000075495 ) ) ;
#2185=CARTESIAN_POINT ( 'NONE',  ( -27.98076211353308551, 49.90833333333318933, -3.845299461620869330 ) ) ;
#2191=ORIENTED_EDGE ( 'NONE', *, *, #9063, .F. ) ;
#2197=EDGE_CURVE ( 'NONE', #5599, #9687, #5106, .T. ) ;
#2199=CARTESIAN_POINT ( 'NONE',  ( -27.60187600103308370, 53.04374999904394627, -5.000000000000103029 ) ) ;
#2205=CARTESIAN_POINT ( 'NONE',  ( -23.98076211353314235, 54.25416666475469185, -3.845299461620867554 ) ) ;
#2210=CARTESIAN_POINT ( 'NONE',  ( -24.35964822603314417, 51.99374999904394201, -5.000000000000103029 ) ) ;
#2212=CARTESIAN_POINT ( 'NONE',  ( -27.60187600103308370, 50.76874999904395480, -5.000000000000103029 ) ) ;
#2216=VECTOR ( 'NONE', #1431, 1000.000000000000000 ) ;
#2219=CARTESIAN_POINT ( 'NONE',  ( -25.98076211353311393, 53.78749999808803040, -7.000000000000072831 ) ) ;
#2225=ORIENTED_EDGE ( 'NONE', *, *, #8168, .F. ) ;
#2230=EDGE_CURVE ( 'NONE', #5764, #10877, #10126, .T. ) ;
#2234=CARTESIAN_POINT ( 'NONE',  ( -25.98076211353311393, 52.38749999808803182, -7.309401076758571314 ) ) ;
#2237=DIRECTION ( 'NONE',  ( 0.000000000000000000, 1.000000000000000000, 0.000000000000000000 ) ) ;
#2239=VERTEX_POINT ( 'NONE', #1628 ) ;
#2244=DIRECTION ( 'NONE',  ( 0.000000000000000000, 1.000000000000000000, 0.000000000000000000 ) ) ;
#2257=CARTESIAN_POINT ( 'NONE',  ( -23.98076211353314235, 51.59999999999985931, -5.000000000000103029 ) ) ;
#2258=CARTESIAN_POINT ( 'NONE',  ( -27.60187600103308370, 51.46874999904395054, -5.000000000000103029 ) ) ;
#2269=DIRECTION ( 'NONE',  ( 0.000000000000000000, 0.000000000000000000, 1.000000000000000000 ) ) ;
#2270=CARTESIAN_POINT ( 'NONE',  ( -25.98076211353310683, 54.44374999904394485, -3.128098921329806714 ) ) ;
#2273=CARTESIAN_POINT ( 'NONE',  ( -25.17020516978313083, 54.03541666571061342, -6.403925809002825709 ) ) ;
#2289=CARTESIAN_POINT ( 'NONE',  ( -27.98076211353308551, 50.40416666475469754, -6.154700538379338504 ) ) ;
#2291=CARTESIAN_POINT ( 'NONE',  ( -27.98076211353308551, 51.22083333142136752, -3.845299461620869330 ) ) ;
#2292=VERTEX_POINT ( 'NONE', #1679 ) ;
#2293=( BOUNDED_CURVE ( )  B_SPLINE_CURVE ( 2, ( #1350, #2808, #5408, #7177, #2972, #6346, #7966, #341, #7023 ),
 .UNSPECIFIED., .F., .T. ) 
 B_SPLINE_CURVE_WITH_KNOTS ( ( 3, 2, 2, 2, 3 ),
 ( 0.4166666666666666852, 0.4259259259259259300, 0.4444444444444444198, 0.4629629629629629650, 0.4722222222222222099 ),
 .UNSPECIFIED. ) 
 CURVE ( )  GEOMETRIC_REPRESENTATION_ITEM ( )  RATIONAL_B_SPLINE_CURVE ( ( 0.9330127018922194093, 0.9330127018922195203, 1.000000000000000000, 0.8660254037844387076, 1.000000000000000000, 0.8660254037844387076, 1.000000000000000000, 0.9330127018922194093, 0.9330127018922194093 ) ) 
 REPRESENTATION_ITEM ( '' )  );
#2305=FACE_OUTER_BOUND ( 'NONE', #8005, .T. ) ;
#2307=APPLICATION_CONTEXT ( 'automotive_design' ) ;
#2308=DIRECTION ( 'NONE',  ( 2.775557561562891351E-17, 1.000000000000000000, -8.326672684688671588E-17 ) ) ;
#2310=CARTESIAN_POINT ( 'NONE',  ( -27.60187600103308014, 55.20208333237728482, -4.064049460664955760 ) ) ;
#2317=CARTESIAN_POINT ( 'NONE',  ( -27.60187600103308725, 53.62708333237728198, -4.064049460664955760 ) ) ;
#2319=CARTESIAN_POINT ( 'NONE',  ( -23.98076211353314235, 50.19999999999986073, -5.000000000000103029 ) ) ;
#2321=CARTESIAN_POINT ( 'NONE',  ( -27.60187600103308014, 55.08541666571061057, -5.935950539335252074 ) ) ;
#2335=CARTESIAN_POINT ( 'NONE',  ( -27.98076211353308551, 51.92083333142137036, -3.845299461620869330 ) ) ;
#2338=ORIENTED_EDGE ( 'NONE', *, *, #2197, .T. ) ;
#2346=CARTESIAN_POINT ( 'NONE',  ( -26.85260690424861707, 57.49300631261340300, -3.199128986994839607 ) ) ;
#2349=( BOUNDED_CURVE ( )  B_SPLINE_CURVE ( 2, ( #10497, #7996, #8883, #4451, #2838, #1213, #9547, #6209, #2887 ),
 .UNSPECIFIED., .F., .F. ) 
 B_SPLINE_CURVE_WITH_KNOTS ( ( 3, 2, 2, 2, 3 ),
 ( 0.08333333333333338422, 0.09259259259259258745, 0.1111111111111111049, 0.1296296296296296224, 0.1388888888888888951 ),
 .UNSPECIFIED. ) 
 CURVE ( )  GEOMETRIC_REPRESENTATION_ITEM ( )  RATIONAL_B_SPLINE_CURVE ( ( 0.9330127018922194093, 0.9330127018922197424, 1.000000000000000000, 0.8660254037844387076, 1.000000000000000000, 0.8660254037844387076, 1.000000000000000000, 0.9330127018922191873, 0.9330127018922192983 ) ) 
 REPRESENTATION_ITEM ( '' )  );
#2351=CARTESIAN_POINT ( 'NONE',  ( -26.98076211353309972, 55.24583333142137320, -6.732050807568954909 ) ) ;
#2359=CARTESIAN_POINT ( 'NONE',  ( -25.17020516978313083, 55.37708333237728198, -3.596074190997380349 ) ) ;
#2361=CARTESIAN_POINT ( 'NONE',  ( -25.98076211353311038, 61.49999999999985789, -8.500000000000694556 ) ) ;
#2367=CARTESIAN_POINT ( 'NONE',  ( -26.79131905728310059, 52.75208333237728198, -6.403925809002825709 ) ) ;
#2369=CARTESIAN_POINT ( 'NONE',  ( -23.98076211353314235, 52.24166666666653924, -3.845299461620867554 ) ) ;
#2370=VERTEX_POINT ( 'NONE', #9066 ) ;
#2371=CARTESIAN_POINT ( 'NONE',  ( -25.98076211353311393, 55.66874999904395338, -6.871901078670400231 ) ) ;
#2375=CARTESIAN_POINT ( 'NONE',  ( -25.98076211353311038, 61.49999999999985789, -5.000000000000102141 ) ) ;
#2387=CARTESIAN_POINT ( 'NONE',  ( -23.98076211353314235, 52.91249999808803040, -5.000000000000103029 ) ) ;
#2398=EDGE_CURVE ( 'NONE', #10879, #8683, #9078, .T. ) ;
#2417=EDGE_CURVE ( 'NONE', #7830, #9083, #4094, .T. ) ;
#2420=CARTESIAN_POINT ( 'NONE',  ( -27.60187600103308370, 55.14374999904394059, -5.000000000000103029 ) ) ;
#2427=CARTESIAN_POINT ( 'NONE',  ( -27.60187600103308725, 50.30208333237727913, -4.064049460664955760 ) ) ;
#2428=CARTESIAN_POINT ( 'NONE',  ( -24.35964822603314772, 53.16041666571062052, -4.064049460664953983 ) ) ;
#2432=CARTESIAN_POINT ( 'NONE',  ( -23.98076211353314235, 52.99999999999986500, -5.000000000000103029 ) ) ;
#2436=VERTEX_POINT ( 'NONE', #735 ) ;
#2451=CARTESIAN_POINT ( 'NONE',  ( -24.98076211353313170, 55.59583333142136752, -3.267949192431250705 ) ) ;
#2455=ORIENTED_EDGE ( 'NONE', *, *, #6340, .F. ) ;
#2466=CARTESIAN_POINT ( 'NONE',  ( -24.98076211353213694, 57.99999999999985789, -9.000000000000701661 ) ) ;
#2471=ORIENTED_EDGE ( 'NONE', *, *, #10105, .T. ) ;
#2473=CARTESIAN_POINT ( 'NONE',  ( -25.98076211353311393, 52.12499999999985079, -3.000000000000132339 ) ) ;
#2479=CARTESIAN_POINT ( 'NONE',  ( -27.60187600103308014, 51.41041666571062052, -5.935950539335252074 ) ) ;
#2486=CARTESIAN_POINT ( 'NONE',  ( -27.60187600103308725, 54.38541666571060773, -5.935950539335252074 ) ) ;
#2487=CARTESIAN_POINT ( 'NONE',  ( -25.17020516978313083, 53.10208333237728340, -3.596074190997380349 ) ) ;
#2489=CARTESIAN_POINT ( 'NONE',  ( -25.98076211353311393, 51.07499999999986784, -7.309401076758571314 ) ) ;
#2490=EDGE_LOOP ( 'NONE', ( #9650, #9091 ) ) ;
#2504=CARTESIAN_POINT ( 'NONE',  ( -24.98076211353312814, 55.82916666475470180, -6.732050807568954909 ) ) ;
#2507=CARTESIAN_POINT ( 'NONE',  ( -27.98076211353308551, 50.46249999808803466, -5.000000000000103029 ) ) ;
#2508=VERTEX_POINT ( 'NONE', #7414 ) ;
#2510=VERTEX_POINT ( 'NONE', #4929 ) ;
#2527=ADVANCED_FACE ( 'NONE', ( #10030, #5804 ), #9190, .F. ) ;
#2528=CYLINDRICAL_SURFACE ( 'NONE', #1346, 1.000000000000972333 ) ;
#2530=CARTESIAN_POINT ( 'NONE',  ( -25.98076211353311038, 59.49999999999985789, -5.000000000000102141 ) ) ;
#2531=CARTESIAN_POINT ( 'NONE',  ( -25.17020516978313083, 54.50208333237728198, -3.596074190997380349 ) ) ;
#2533=CARTESIAN_POINT ( 'NONE',  ( -25.71414987012866504, 57.02732617680999994, -3.014027881576975876 ) ) ;
#2540=CARTESIAN_POINT ( 'NONE',  ( -25.98076211353310683, 53.21874999904395054, -3.128098921329806714 ) ) ;
#2544=CARTESIAN_POINT ( 'NONE',  ( -25.98076211353311393, 53.87499999999985789, -7.309401076758571314 ) ) ;
#2547=VERTEX_POINT ( 'NONE', #5205 ) ;
#2561=AXIS2_PLACEMENT_3D ( 'NONE', #1379, #3976, #10756 ) ;
#2563=CARTESIAN_POINT ( 'NONE',  ( -23.98076211353314235, 55.71249999808803466, -5.000000000000103029 ) ) ;
#2566=CARTESIAN_POINT ( 'NONE',  ( -25.98076211353311393, 52.12499999999985079, -3.000000000000132783 ) ) ;
#2570=ORIENTED_EDGE ( 'NONE', *, *, #1797, .T. ) ;
#2577=CARTESIAN_POINT ( 'NONE',  ( -25.98076211353311393, 52.69374999904394485, -6.871901078670400231 ) ) ;
#2581=AXIS2_PLACEMENT_3D ( 'NONE', #2597, #2674, #3609 ) ;
#2595=CARTESIAN_POINT ( 'NONE',  ( -24.35964822603314772, 53.27708333237728056, -5.935950539335252074 ) ) ;
#2597=CARTESIAN_POINT ( 'NONE',  ( -25.98076211353311393, 49.49999999999986500, -5.000000000000103029 ) ) ;
#2603=CARTESIAN_POINT ( 'NONE',  ( -27.98076211353308551, 54.10833333333319928, -3.845299461620869330 ) ) ;
#2604=CARTESIAN_POINT ( 'NONE',  ( -26.79131905728310059, 53.86041666571061626, -3.596074190997381237 ) ) ;
#2605=CARTESIAN_POINT ( 'NONE',  ( -25.98076211353311393, 55.27499999999985647, -7.000000000000072831 ) ) ;
#2606=CIRCLE ( 'NONE', #4010, 4.000000000000600409 ) ;
#2608=CARTESIAN_POINT ( 'NONE',  ( -23.98076211353314235, 53.05833333333319501, -6.154700538379337615 ) ) ;
#2613=ADVANCED_FACE ( 'NONE', ( #1811 ), #4484, .T. ) ;
#2616=ORIENTED_EDGE ( 'NONE', *, *, #5161, .T. ) ;
#2619=CARTESIAN_POINT ( 'NONE',  ( -24.98076211353313170, 54.28333333333319644, -3.267949192431250705 ) ) ;
#2626=CARTESIAN_POINT ( 'NONE',  ( -26.79131905728310059, 50.36041666571060915, -3.596074190997381237 ) ) ;
#2629=CARTESIAN_POINT ( 'NONE',  ( -25.98076211353415843, 59.00000000000900968, -2.999999999996041389 ) ) ;
#2638=CARTESIAN_POINT ( 'NONE',  ( -24.98076211353213694, 58.13434381516401572, -6.732050807568384698 ) ) ;
#2641=CARTESIAN_POINT ( 'NONE',  ( -26.79131905728310059, 50.18541666571061199, -3.596074190997381237 ) ) ;
#2642=VECTOR ( 'NONE', #8700, 1000.000000000000000 ) ;
#2646=VERTEX_POINT ( 'NONE', #10195 ) ;
#2655=CARTESIAN_POINT ( 'NONE',  ( -25.17020516978313083, 53.80208333237728624, -3.596074190997380349 ) ) ;
#2661=CARTESIAN_POINT ( 'NONE',  ( -26.98076211353309972, 50.43333333333319501, -6.732050807568954909 ) ) ;
#2663=CARTESIAN_POINT ( 'NONE',  ( -24.35964822603314772, 53.33541666571061768, -4.064049460664953983 ) ) ;
#2674=DIRECTION ( 'NONE',  ( 0.000000000000000000, 1.000000000000000000, 0.000000000000000000 ) ) ;
#2679=CARTESIAN_POINT ( 'NONE',  ( -27.98076211353308551, 55.36249999808803324, -5.000000000000103029 ) ) ;
#2691=CARTESIAN_POINT ( 'NONE',  ( -27.60187600103308370, 50.06874999904395196, -5.000000000000103029 ) ) ;
#2692=AXIS2_PLACEMENT_3D ( 'NONE', #5915, #9298, #6746 ) ;
#2701=FACE_OUTER_BOUND ( 'NONE', #9834, .T. ) ;
#2704=CARTESIAN_POINT ( 'NONE',  ( -27.69734467828301305, 55.55430429566774819, -4.173301533939525854 ) ) ;
#2705=CARTESIAN_POINT ( 'NONE',  ( -27.60187600103308014, 54.21041666571061768, -5.935950539335252074 ) ) ;
#2708=CARTESIAN_POINT ( 'NONE',  ( -25.10838757727078630, 57.49417738710737069, -3.199400465621848433 ) ) ;
#2715=CARTESIAN_POINT ( 'NONE',  ( -27.60187600103308725, 53.10208333237727629, -4.064049460664955760 ) ) ;
#2717=CARTESIAN_POINT ( 'NONE',  ( -24.98076211353313170, 50.78333333333319644, -3.267949192431250705 ) ) ;
#2719=CARTESIAN_POINT ( 'NONE',  ( -26.98076211353309972, 54.16666666666652930, -3.267949192431252037 ) ) ;
#2728=CARTESIAN_POINT ( 'NONE',  ( -23.98076211353314235, 54.45833333333320070, -6.154700538379337615 ) ) ;
#2731=CARTESIAN_POINT ( 'NONE',  ( -27.60187600103308370, 52.34374999904394343, -5.000000000000103029 ) ) ;
#2732=CARTESIAN_POINT ( 'NONE',  ( -25.98076211353311393, 54.48749999808803324, -7.000000000000072831 ) ) ;
#2744=CARTESIAN_POINT ( 'NONE',  ( -27.60187600103308014, 50.71041666571061768, -5.935950539335252074 ) ) ;
#2748=EDGE_CURVE ( 'NONE', #8872, #9873, #1188, .T. ) ;
#2749=ORIENTED_EDGE ( 'NONE', *, *, #10749, .F. ) ;
#2750=ORIENTED_EDGE ( 'NONE', *, *, #8713, .T. ) ;
#2751=AXIS2_PLACEMENT_3D ( 'NONE', #4502, #6320, #9712 ) ;
#2753=FACE_OUTER_BOUND ( 'NONE', #2121, .T. ) ;
#2758=CARTESIAN_POINT ( 'NONE',  ( -26.79131905728310059, 52.05208333237728624, -6.403925809002825709 ) ) ;
#2762=EDGE_CURVE ( 'NONE', #2239, #2510, #2801, .T. ) ;
#2773=CARTESIAN_POINT ( 'NONE',  ( -23.98076211353314235, 55.01249999808803182, -5.000000000000103029 ) ) ;
#2787=EDGE_CURVE ( 'NONE', #276, #4873, #7366, .T. ) ;
#2790=CARTESIAN_POINT ( 'NONE',  ( -25.98076211353311393, 51.81874999904394485, -3.128098921329806714 ) ) ;
#2801=B_SPLINE_CURVE_WITH_KNOTS ( 'NONE', 3,
 ( #2982, #4697, #8912, #1302, #9854, #10639, #455, #1358, #7242, #8805 ),
 .UNSPECIFIED., .F., .F.,
 ( 4, 2, 2, 2, 4 ),
 ( 0.000000000000000000, 0.0003977372743948460413, 0.0007954745487896920826, 0.001193211823184538124, 0.001590949097579384165 ),
 .UNSPECIFIED. ) ;
#2803=CARTESIAN_POINT ( 'NONE',  ( -27.60187600103308014, 54.21041666571061768, -5.935950539335252074 ) ) ;
#2808=CARTESIAN_POINT ( 'NONE',  ( -25.44486372867087098, 52.76876073720499249, -3.000000000000133227 ) ) ;
#2818=CARTESIAN_POINT ( 'NONE',  ( -25.98076211353311749, 56.99999999999886313, -3.000000000000122569 ) ) ;
#2819=EDGE_CURVE ( 'NONE', #6817, #7809, #3179, .T. ) ;
#2820=FILL_AREA_STYLE_COLOUR ( '', #8846 ) ;
#2824=CARTESIAN_POINT ( 'NONE',  ( -25.98076211353311038, 60.99999999999985789, -9.000000000000701661 ) ) ;
#2833=CARTESIAN_POINT ( 'NONE',  ( -24.35964822603314772, 51.35208333237728340, -5.935950539335252074 ) ) ;
#2838=CARTESIAN_POINT ( 'NONE',  ( -23.98076211353314235, 50.81249999808803608, -5.000000000000103029 ) ) ;
#2847=CARTESIAN_POINT ( 'NONE',  ( -25.98076211353311393, 49.49999999999986500, -7.000000000000074607 ) ) ;
#2848=CARTESIAN_POINT ( 'NONE',  ( -24.35964822603314417, 51.99374999904394201, -5.000000000000103029 ) ) ;
#2851=CARTESIAN_POINT ( 'NONE',  ( -25.98076211353311393, 54.83749999808803466, -3.000000000000132339 ) ) ;
#2859=CARTESIAN_POINT ( 'NONE',  ( -23.98076211353314235, 49.49999999999986500, -5.000000000000103029 ) ) ;
#2862=CARTESIAN_POINT ( 'NONE',  ( -26.24690541728881499, 58.97268535620265340, -6.985987684901640904 ) ) ;
#2871=CARTESIAN_POINT ( 'NONE',  ( -25.98076211353311393, 49.49999999999986500, -7.000000000000074607 ) ) ;
#2878=EDGE_CURVE ( 'NONE', #2239, #8562, #10127, .T. ) ;
#2879=CARTESIAN_POINT ( 'NONE',  ( -25.98076211353311393, 55.18749999808803608, -7.000000000000072831 ) ) ;
#2880=CARTESIAN_POINT ( 'NONE',  ( -25.98076211353311393, 53.78749999808803040, -7.000000000000072831 ) ) ;
#2882=CARTESIAN_POINT ( 'NONE',  ( -27.60187600103308370, 54.44374999904394485, -5.000000000000103029 ) ) ;
#2887=CARTESIAN_POINT ( 'NONE',  ( -25.98076211353311393, 50.98749999808804034, -7.000000000000073719 ) ) ;
#2895=CARTESIAN_POINT ( 'NONE',  ( -24.35964822603314417, 50.41874999904395338, -5.000000000000103029 ) ) ;
#2899=CARTESIAN_POINT ( 'NONE',  ( -26.79131905728310059, 51.76041666571061484, -3.596074190997381237 ) ) ;
#2908=EDGE_CURVE ( 'NONE', #3474, #10992, #9421, .T. ) ;
#2911=CARTESIAN_POINT ( 'NONE',  ( -27.60187600103308014, 53.62708333237728908, -4.064049460664955760 ) ) ;
#2923=CARTESIAN_POINT ( 'NONE',  ( -25.98076211353311393, 50.37499999999987210, -7.000000000000073719 ) ) ;
#2924=CARTESIAN_POINT ( 'NONE',  ( -25.44486372867087098, 49.64373926088289579, -7.000000000000072831 ) ) ;
#2928=CIRCLE ( 'NONE', #3092, 1.999999999999971356 ) ;
#2936=CARTESIAN_POINT ( 'NONE',  ( -25.98076211353311393, 52.82499999999986784, -3.000000000000132339 ) ) ;
#2938=CARTESIAN_POINT ( 'NONE',  ( -25.98076211353311393, 52.51874999904395480, -3.128098921329806714 ) ) ;
#2945=CARTESIAN_POINT ( 'NONE',  ( -25.98076211353311038, 61.49999999999985789, -5.000000000000102141 ) ) ;
#2954=CARTESIAN_POINT ( 'NONE',  ( -24.35964822603314772, 54.85208333237728340, -5.935950539335252074 ) ) ;
#2964=ADVANCED_FACE ( 'NONE', ( #9117 ), #9962, .T. ) ;
#2967=EDGE_CURVE ( 'NONE', #9280, #8338, #724, .T. ) ;
#2972=CARTESIAN_POINT ( 'NONE',  ( -23.98076211353314235, 52.91249999808803040, -5.000000000000103029 ) ) ;
#2981=PRODUCT_DEFINITION_FORMATION_WITH_SPECIFIED_SOURCE ( 'ANY', '', #7066, .NOT_KNOWN. ) ;
#2982=CARTESIAN_POINT ( 'NONE',  ( -24.98076211353213694, 57.99999999999985789, -6.732050807568384698 ) ) ;
#2992=CARTESIAN_POINT ( 'NONE',  ( -25.98076211353311393, 52.03749999808803750, -3.000000000000132339 ) ) ;
#2995=CARTESIAN_POINT ( 'NONE',  ( -27.60187600103308014, 53.10208333237727629, -4.064049460664955760 ) ) ;
#2998=VECTOR ( 'NONE', #767, 1000.000000000000000 ) ;
#3004=CARTESIAN_POINT ( 'NONE',  ( -27.78268512908116961, 55.49961679590672503, -4.132201955500060642 ) ) ;
#3005=CARTESIAN_POINT ( 'NONE',  ( -25.17020516978313083, 51.00208333237728198, -3.596074190997380349 ) ) ;
#3014=VERTEX_POINT ( 'NONE', #8520 ) ;
#3020=CARTESIAN_POINT ( 'NONE',  ( -27.98076211353308551, 51.22083333142136752, -3.845299461620869330 ) ) ;
#3025=ADVANCED_FACE ( 'NONE', ( #1800 ), #9931, .T. ) ;
#3041=CARTESIAN_POINT ( 'NONE',  ( -25.44486372867087454, 51.74373926088290432, -7.000000000000073719 ) ) ;
#3042=CARTESIAN_POINT ( 'NONE',  ( -26.79131905728310059, 53.62708333237727487, -6.403925809002825709 ) ) ;
#3047=CARTESIAN_POINT ( 'NONE',  ( -23.98076211353314235, 54.31249999808803608, -5.000000000000103029 ) ) ;
#3051=CARTESIAN_POINT ( 'NONE',  ( -25.98076211353310683, 50.41874999904394627, -3.128098921329806714 ) ) ;
#3053=CARTESIAN_POINT ( 'NONE',  ( -25.98076211353310683, 50.24374999904394912, -3.128098921329806714 ) ) ;
#3056=ORIENTED_EDGE ( 'NONE', *, *, #2967, .F. ) ;
#3066=CARTESIAN_POINT ( 'NONE',  ( -23.98076211353314235, 50.87083333142136610, -6.154700538379337615 ) ) ;
#3070=ADVANCED_FACE ( 'NONE', ( #6041 ), #7882, .T. ) ;
#3079=DIRECTION ( 'NONE',  ( 0.000000000000000000, 1.000000000000000000, 0.000000000000000000 ) ) ;
#3082=CARTESIAN_POINT ( 'NONE',  ( -25.98076211353311393, 55.18749999808803608, -7.000000000000072831 ) ) ;
#3087=CARTESIAN_POINT ( 'NONE',  ( -23.98076211353314235, 52.15416666475469754, -3.845299461620867554 ) ) ;
#3090=CARTESIAN_POINT ( 'NONE',  ( -26.51666049839535688, 51.10626073911683420, -7.000000000000074607 ) ) ;
#3091=CARTESIAN_POINT ( 'NONE',  ( -26.79131905728310059, 51.35208333237728340, -6.403925809002825709 ) ) ;
#3092=AXIS2_PLACEMENT_3D ( 'NONE', #8153, #5756, #9039 ) ;
#3100=CARTESIAN_POINT ( 'NONE',  ( -25.98076211353310683, 54.79374999904395338, -6.871901078670399343 ) ) ;
#3103=CARTESIAN_POINT ( 'NONE',  ( -27.60187600103308370, 53.56874999904395196, -5.000000000000103029 ) ) ;
#3119=CARTESIAN_POINT ( 'NONE',  ( -25.98076211353311393, 53.43749999808803608, -2.690598923241634743 ) ) ;
#3120=CARTESIAN_POINT ( 'NONE',  ( -25.98076211353310683, 53.52499999999986358, -3.000000000000132339 ) ) ;
#3123=ORIENTED_EDGE ( 'NONE', *, *, #8444, .T. ) ;
#3128=CARTESIAN_POINT ( 'NONE',  ( -26.48810847200994090, 57.12842764990476496, -3.061534065193112220 ) ) ;
#3140=CARTESIAN_POINT ( 'NONE',  ( -25.98076211353311393, 51.64374999904395480, -3.128098921329806714 ) ) ;
#3143=ORIENTED_EDGE ( 'NONE', *, *, #10749, .T. ) ;
#3147=CARTESIAN_POINT ( 'NONE',  ( -25.98076211353311393, 49.49999999999986500, -5.000000000000103029 ) ) ;
#3151=CARTESIAN_POINT ( 'NONE',  ( -27.60187600103308370, 51.46874999904395054, -5.000000000000103029 ) ) ;
#3154=CARTESIAN_POINT ( 'NONE',  ( -24.98076211353313170, 50.08333333333319359, -3.267949192431250705 ) ) ;
#3157=ORIENTED_EDGE ( 'NONE', *, *, #5699, .T. ) ;
#3170=CARTESIAN_POINT ( 'NONE',  ( -26.98076211353309972, 50.57916666475469469, -3.267949192431252037 ) ) ;
#3172=CARTESIAN_POINT ( 'NONE',  ( -25.98076211353311038, 59.49999999999985789, -5.000000000000102141 ) ) ;
#3178=DIRECTION ( 'NONE',  ( 0.000000000000000000, 1.000000000000000000, 0.000000000000000000 ) ) ;
#3179=( BOUNDED_CURVE ( )  B_SPLINE_CURVE ( 1, ( #7134, #10529 ),
 .UNSPECIFIED., .F., .F. ) 
 B_SPLINE_CURVE_WITH_KNOTS ( ( 2, 2 ),
 ( 0.000000000000000000, 1.000000000000000000 ),
 .UNSPECIFIED. ) 
 CURVE ( )  GEOMETRIC_REPRESENTATION_ITEM ( )  RATIONAL_B_SPLINE_CURVE ( ( 0.9343183815700366601, 0.9343183815700366601 ) ) 
 REPRESENTATION_ITEM ( '' )  );
#3184=VERTEX_POINT ( 'NONE', #5703 ) ;
#3185=CARTESIAN_POINT ( 'NONE',  ( -25.98076211353311393, 49.49999999999986500, -5.000000000000103029 ) ) ;
#3192=CARTESIAN_POINT ( 'NONE',  ( -26.79131905728310059, 49.95208333237728482, -6.403925809002825709 ) ) ;
#3199=CARTESIAN_POINT ( 'NONE',  ( -25.17020516978313083, 50.01041666571061484, -6.403925809002825709 ) ) ;
#3200=CARTESIAN_POINT ( 'NONE',  ( -26.79131905728310059, 51.58541666571061768, -3.596074190997381237 ) ) ;
#3203=CARTESIAN_POINT ( 'NONE',  ( -26.98076211353309972, 50.43333333333319501, -6.732050807568954909 ) ) ;
#3206=CARTESIAN_POINT ( 'NONE',  ( -25.17020516978313083, 55.37708333237728198, -3.596074190997380349 ) ) ;
#3222=CARTESIAN_POINT ( 'NONE',  ( -23.98076211353314235, 52.15416666475470464, -3.845299461620867554 ) ) ;
#3231=EDGE_CURVE ( 'NONE', #8338, #4274, #5041, .T. ) ;
#3241=CARTESIAN_POINT ( 'NONE',  ( -25.98076211353310683, 55.53749999808803040, -3.000000000000132339 ) ) ;
#3243=ORIENTED_EDGE ( 'NONE', *, *, #5785, .F. ) ;
#3246=CARTESIAN_POINT ( 'NONE',  ( -25.98076211353311393, 49.49999999999986500, -3.000000000000131894 ) ) ;
#3250=CARTESIAN_POINT ( 'NONE',  ( -25.98076211353311393, 55.66874999904395338, -6.871901078670400231 ) ) ;
#3256=CARTESIAN_POINT ( 'NONE',  ( -26.98076211353309972, 53.93333333333319501, -6.732050807568954909 ) ) ;
#3257=CARTESIAN_POINT ( 'NONE',  ( -27.60187600103308370, 51.64374999904394770, -5.000000000000103029 ) ) ;
#3258=CARTESIAN_POINT ( 'NONE',  ( -24.35964822603314772, 53.97708333237729050, -5.935950539335252074 ) ) ;
#3260=CARTESIAN_POINT ( 'NONE',  ( -26.98076211353309972, 52.06666666666653498, -3.267949192431252037 ) ) ;
#3274=VECTOR ( 'NONE', #8714, 1000.000000000000000 ) ;
#3275=CARTESIAN_POINT ( 'NONE',  ( -24.35964822603314772, 50.53541666571060631, -4.064049460664953983 ) ) ;
#3278=CARTESIAN_POINT ( 'NONE',  ( -24.98076211353313170, 54.19583333142136894, -3.267949192431250705 ) ) ;
#3286=AXIS2_PLACEMENT_3D ( 'NONE', #186, #7130, #1920 ) ;
#3295=CONICAL_SURFACE ( 'NONE', #8254, 3.500000000000591971, 0.7853981633974560506 ) ;
#3298=CARTESIAN_POINT ( 'NONE',  ( -24.98076211353313170, 51.39583333142136468, -3.267949192431250705 ) ) ;
#3309=CARTESIAN_POINT ( 'NONE',  ( -25.17020516978313083, 51.23541666571061626, -6.403925809002825709 ) ) ;
#3316=CARTESIAN_POINT ( 'NONE',  ( -25.17020516978313083, 52.81041666571061199, -6.403925809002825709 ) ) ;
#3318=CARTESIAN_POINT ( 'NONE',  ( -26.79131905728310059, 54.85208333237729050, -6.403925809002825709 ) ) ;
#3321=CARTESIAN_POINT ( 'NONE',  ( -27.98076211353308551, 52.64999999999986358, -5.000000000000103029 ) ) ;
#3324=VERTEX_POINT ( 'NONE', #5866 ) ;
#3327=CARTESIAN_POINT ( 'NONE',  ( -25.98076211353311393, 59.49999999999985789, -3.000000000000131894 ) ) ;
#3332=VECTOR ( 'NONE', #7557, 1000.000000000000000 ) ;
#3338=CARTESIAN_POINT ( 'NONE',  ( -23.98076211353314235, 55.65416666475469754, -3.845299461620867554 ) ) ;
#3341=CARTESIAN_POINT ( 'NONE',  ( -24.98076211353313170, 53.58333333333320070, -3.267949192431250705 ) ) ;
#3342=ORIENTED_EDGE ( 'NONE', *, *, #7314, .F. ) ;
#3344=ORIENTED_EDGE ( 'NONE', *, *, #10382, .F. ) ;
#3366=CARTESIAN_POINT ( 'NONE',  ( -25.98076211353311393, 49.49999999999986500, -3.000000000000131894 ) ) ;
#3367=CARTESIAN_POINT ( 'NONE',  ( -27.60187600103308014, 53.62708333237728908, -4.064049460664955760 ) ) ;
#3370=CARTESIAN_POINT ( 'NONE',  ( -25.98076211353311038, 61.49999999999985789, -5.000000000000102141 ) ) ;
#3372=ORIENTED_EDGE ( 'NONE', *, *, #2762, .F. ) ;
#3374=CARTESIAN_POINT ( 'NONE',  ( -26.98076211353309972, 54.16666666666652930, -3.267949192431252037 ) ) ;
#3376=CARTESIAN_POINT ( 'NONE',  ( -25.98076211353310683, 54.61874999904394912, -3.128098921329806714 ) ) ;
#3379=CARTESIAN_POINT ( 'NONE',  ( -23.98076211353314235, 53.69999999999986784, -5.000000000000103029 ) ) ;
#3382=ADVANCED_FACE ( 'NONE', ( #5919 ), #3295, .T. ) ;
#3393=CARTESIAN_POINT ( 'NONE',  ( -25.98076211353311038, 59.49999999999985789, -9.000000000000701661 ) ) ;
#3394=CARTESIAN_POINT ( 'NONE',  ( -26.79131905728310059, 51.06041666571061199, -3.596074190997381237 ) ) ;
#3399=ORIENTED_EDGE ( 'NONE', *, *, #1796, .F. ) ;
#3404=EDGE_CURVE ( 'NONE', #1738, #2370, #4004, .T. ) ;
#3407=CARTESIAN_POINT ( 'NONE',  ( -25.17020516978313083, 52.40208333237728766, -3.596074190997380349 ) ) ;
#3421=CARTESIAN_POINT ( 'NONE',  ( -25.98076211353310683, 55.53749999808803040, -3.000000000000132339 ) ) ;
#3424=CARTESIAN_POINT ( 'NONE',  ( -25.17020516978313083, 54.03541666571061342, -6.403925809002825709 ) ) ;
#3432=( BOUNDED_CURVE ( )  B_SPLINE_CURVE ( 2, ( #5491, #1938, #311, #3598, #2773, #7095, #4605, #7987, #2879 ),
 .UNSPECIFIED., .F., .F. ) 
 B_SPLINE_CURVE_WITH_KNOTS ( ( 3, 2, 2, 2, 3 ),
 ( 0.7500000000000000000, 0.7592592592592593004, 0.7777777777777777901, 0.7962962962962962798, 0.8055555555555555802 ),
 .UNSPECIFIED. ) 
 CURVE ( )  GEOMETRIC_REPRESENTATION_ITEM ( )  RATIONAL_B_SPLINE_CURVE ( ( 0.9330127018922194093, 0.9330127018922194093, 1.000000000000000000, 0.8660254037844387076, 1.000000000000000000, 0.8660254037844387076, 1.000000000000000000, 0.9330127018922189652, 0.9330127018922194093 ) ) 
 REPRESENTATION_ITEM ( '' )  );
#3433=CARTESIAN_POINT ( 'NONE',  ( -25.17020516978313083, 52.57708333237728482, -3.596074190997380349 ) ) ;
#3438=CARTESIAN_POINT ( 'NONE',  ( -27.98076211353308551, 51.30833333333320212, -3.845299461620869330 ) ) ;
#3451=CARTESIAN_POINT ( 'NONE',  ( -25.98076211353311393, 50.06874999904394485, -6.871901078670400231 ) ) ;
#3455=CARTESIAN_POINT ( 'NONE',  ( -26.79131905728310059, 50.12708333237728198, -6.403925809002825709 ) ) ;
#3458=CARTESIAN_POINT ( 'NONE',  ( -25.18320465585345502, 58.61672392917972729, -3.163343793118901903 ) ) ;
#3467=CARTESIAN_POINT ( 'NONE',  ( -27.60187600103308370, 50.76874999904395480, -5.000000000000103029 ) ) ;
#3474=VERTEX_POINT ( 'NONE', #10424 ) ;
#3475=CARTESIAN_POINT ( 'NONE',  ( -27.98076211353308551, 51.89166666666653782, -6.154700538379338504 ) ) ;
#3476=VECTOR ( 'NONE', #3178, 1000.000000000000000 ) ;
#3482=CARTESIAN_POINT ( 'NONE',  ( -25.98076211353311393, 54.79374999904395338, -6.871901078670400231 ) ) ;
#3489=CARTESIAN_POINT ( 'NONE',  ( -25.17020516978313083, 52.11041666571060915, -6.403925809002825709 ) ) ;
#3490=CARTESIAN_POINT ( 'NONE',  ( -25.44486372867087809, 50.75626073911681857, -3.000000000000133671 ) ) ;
#3493=CARTESIAN_POINT ( 'NONE',  ( -26.98076211353309972, 54.86666666666653214, -3.267949192431252037 ) ) ;
#3500=SHAPE_DEFINITION_REPRESENTATION ( #6780, #5283 ) ;
#3509=CARTESIAN_POINT ( 'NONE',  ( -27.98076211353308551, 54.66249999808803040, -5.000000000000103029 ) ) ;
#3524=CARTESIAN_POINT ( 'NONE',  ( -27.60187600103308014, 50.82708333237729192, -4.064049460664955760 ) ) ;
#3537=CARTESIAN_POINT ( 'NONE',  ( -26.51666049839534978, 52.79373926088290148, -3.000000000000133227 ) ) ;
#3539=CARTESIAN_POINT ( 'NONE',  ( -25.98076211353311393, 53.74374999904394912, -3.128098921329806714 ) ) ;
#3547=CARTESIAN_POINT ( 'NONE',  ( -24.35964822603314772, 55.55208333237727913, -5.935950539335252074 ) ) ;
#3548=DIRECTION ( 'NONE',  ( 0.000000000000000000, 1.000000000000000000, 0.000000000000000000 ) ) ;
#3549=CARTESIAN_POINT ( 'NONE',  ( -25.98076211353311393, 49.49999999999986500, -3.000000000000131894 ) ) ;
#3550=CARTESIAN_POINT ( 'NONE',  ( -27.98076211353308551, 55.39166666666653072, -6.154700538379338504 ) ) ;
#3559=CARTESIAN_POINT ( 'NONE',  ( -23.98076211353314235, 54.39999999999986358, -5.000000000000103029 ) ) ;
#3564=CARTESIAN_POINT ( 'NONE',  ( -24.35964822603314772, 52.75208333237727487, -5.935950539335252074 ) ) ;
#3575=CARTESIAN_POINT ( 'NONE',  ( -25.98076211353311393, 50.59374999904395054, -6.871901078670400231 ) ) ;
#3579=CARTESIAN_POINT ( 'NONE',  ( -26.98076211353408382, 57.99999999999985789, -6.732050807568389139 ) ) ;
#3582=EDGE_CURVE ( 'NONE', #433, #6171, #914, .T. ) ;
#3589=DIRECTION ( 'NONE',  ( -0.9009800080279036782, 0.000000000000000000, 0.4338606056489096585 ) ) ;
#3590=CARTESIAN_POINT ( 'NONE',  ( -26.79131905728310059, 55.55208333237728624, -6.403925809002825709 ) ) ;
#3591=DIRECTION ( 'NONE',  ( 0.000000000000000000, 0.000000000000000000, 1.000000000000000000 ) ) ;
#3598=CARTESIAN_POINT ( 'NONE',  ( -23.98076211353314235, 54.95416666475470180, -3.845299461620867554 ) ) ;
#3606=CARTESIAN_POINT ( 'NONE',  ( -25.98076211353311393, 54.57499999999986073, -7.000000000000072831 ) ) ;
#3608=VERTEX_POINT ( 'NONE', #9696 ) ;
#3609=DIRECTION ( 'NONE',  ( 0.000000000000000000, 0.000000000000000000, 1.000000000000000000 ) ) ;
#3613=CARTESIAN_POINT ( 'NONE',  ( -27.60187600103308014, 52.98541666571061626, -5.935950539335252074 ) ) ;
#3614=DIRECTION ( 'NONE',  ( 0.000000000000000000, 1.000000000000000000, 0.000000000000000000 ) ) ;
#3625=CARTESIAN_POINT ( 'NONE',  ( -24.35964822603314772, 50.36041666571061626, -4.064049460664953983 ) ) ;
#3628=CYLINDRICAL_SURFACE ( 'NONE', #9173, 1.999999999999971356 ) ;
#3638=CARTESIAN_POINT ( 'NONE',  ( -27.78269984933782411, 56.11211482050297406, -4.132232521764788835 ) ) ;
#3650=VECTOR ( 'NONE', #8862, 1000.000000000000000 ) ;
#3653=CARTESIAN_POINT ( 'NONE',  ( -23.98076211353314235, 52.94166666666653498, -3.845299461620867554 ) ) ;
#3664=ADVANCED_FACE ( 'NONE', ( #8082 ), #10533, .T. ) ;
#3670=CARTESIAN_POINT ( 'NONE',  ( -27.60187600103308014, 54.50208333237726777, -4.064049460664955760 ) ) ;
#3672=EDGE_LOOP ( 'NONE', ( #5769, #130 ) ) ;
#3678=CARTESIAN_POINT ( 'NONE',  ( -27.60187600103308370, 50.94374999904394485, -5.000000000000103029 ) ) ;
#3679=( NAMED_UNIT ( * ) SI_UNIT ( $, .STERADIAN. ) SOLID_ANGLE_UNIT ( ) );
#3682=CARTESIAN_POINT ( 'NONE',  ( -25.17020516978313083, 54.73541666571062336, -6.403925809002825709 ) ) ;
#3686=EDGE_CURVE ( 'NONE', #5523, #4738, #8186, .T. ) ;
#3689=LINE ( 'NONE', #1974, #3650 ) ;
#3691=STYLED_ITEM ( 'NONE', ( #1340 ), #3752 ) ;
#3693=CARTESIAN_POINT ( 'NONE',  ( -26.85339429124058697, 58.50531623421669281, -3.199529906863744166 ) ) ;
#3694=CARTESIAN_POINT ( 'NONE',  ( -27.98076211353308551, 52.62083333142137320, -3.845299461620869330 ) ) ;
#3706=CARTESIAN_POINT ( 'NONE',  ( -26.95340920277349284, 57.73396742993422492, -6.748466501715046029 ) ) ;
#3707=CARTESIAN_POINT ( 'NONE',  ( -25.44486372867087809, 52.85626073911682710, -3.000000000000132339 ) ) ;
#3709=CARTESIAN_POINT ( 'NONE',  ( -25.17020516978313083, 52.81041666571061199, -6.403925809002825709 ) ) ;
#3711=CARTESIAN_POINT ( 'NONE',  ( -23.98076211353314235, 54.45833333333320070, -6.154700538379337615 ) ) ;
#3712=ORIENTED_EDGE ( 'NONE', *, *, #703, .T. ) ;
#3720=CARTESIAN_POINT ( 'NONE',  ( -27.78269984933782411, 56.11211482050296695, -4.132232521764788835 ) ) ;
#3721=CARTESIAN_POINT ( 'NONE',  ( -25.17020516978313083, 50.30208333237728624, -3.596074190997380349 ) ) ;
#3724=CARTESIAN_POINT ( 'NONE',  ( -27.60187600103308370, 53.74374999904394201, -5.000000000000103029 ) ) ;
#3735=CARTESIAN_POINT ( 'NONE',  ( -27.60187600103308014, 55.61041666571061626, -5.935950539335252074 ) ) ;
#3739=EDGE_LOOP ( 'NONE', ( #474, #3123, #10175, #6714 ) ) ;
#3747=CARTESIAN_POINT ( 'NONE',  ( -25.98076211353311393, 52.73749999808803324, -3.000000000000132339 ) ) ;
#3749=CARTESIAN_POINT ( 'NONE',  ( -23.98076211353314235, 49.49999999999986500, -5.000000000000103029 ) ) ;
#3752=ADVANCED_BREP_SHAPE_REPRESENTATION ( '', ( #1846, #308 ), #6179 ) ;
#3764=CARTESIAN_POINT ( 'NONE',  ( -27.98076211353308551, 51.24999999999986500, -5.000000000000103029 ) ) ;
#3765=CARTESIAN_POINT ( 'NONE',  ( -27.60187600103308014, 52.98541666571061626, -5.935950539335252074 ) ) ;
#3768=ORIENTED_EDGE ( 'NONE', *, *, #9586, .F. ) ;
#3769=EDGE_LOOP ( 'NONE', ( #4217, #4922, #2338, #587, #8729, #6322, #7664, #8390, #6381, #7736, #7365, #5368, #8945, #9292, #7163, #739, #6491, #4952, #7406, #10035, #4100 ) ) ;
#3770=FACE_OUTER_BOUND ( 'NONE', #2019, .T. ) ;
#3776=CARTESIAN_POINT ( 'NONE',  ( -24.35964822603314772, 49.77708333237728766, -5.935950539335252074 ) ) ;
#3780=CARTESIAN_POINT ( 'NONE',  ( -26.79131905728310059, 53.62708333237727487, -6.403925809002825709 ) ) ;
#3781=EDGE_LOOP ( 'NONE', ( #1827, #1886, #3399 ) ) ;
#3788=( BOUNDED_CURVE ( )  B_SPLINE_CURVE ( 2, ( #8174, #4964, #9902, #6443, #3901, #2291, #1504, #10838, #8220 ),
 .UNSPECIFIED., .F., .F. ) 
 B_SPLINE_CURVE_WITH_KNOTS ( ( 3, 2, 2, 2, 3 ),
 ( 0.1388888888888888951, 0.1481481481481481399, 0.1666666666666666574, 0.1851851851851851749, 0.1944444444444444198 ),
 .UNSPECIFIED. ) 
 CURVE ( )  GEOMETRIC_REPRESENTATION_ITEM ( )  RATIONAL_B_SPLINE_CURVE ( ( 0.9330127018922192983, 0.9330127018922194093, 1.000000000000000000, 0.8660254037844387076, 1.000000000000000000, 0.8660254037844387076, 1.000000000000000000, 0.9330127018922194093, 0.9330127018922192983 ) ) 
 REPRESENTATION_ITEM ( '' )  );
#3791=CARTESIAN_POINT ( 'NONE',  ( -27.98076211353308551, 49.90833333333318933, -3.845299461620869330 ) ) ;
#3798=CARTESIAN_POINT ( 'NONE',  ( -24.35964822603314417, 49.71874999904395054, -5.000000000000103029 ) ) ;
#3799=CARTESIAN_POINT ( 'NONE',  ( -27.98076211353308551, 56.00416666475469896, -6.154700538379338504 ) ) ;
#3805=ORIENTED_EDGE ( 'NONE', *, *, #1740, .T. ) ;
#3811=CARTESIAN_POINT ( 'NONE',  ( -26.48978331829069788, 57.12923484186614331, -6.938092349935781833 ) ) ;
#3813=CARTESIAN_POINT ( 'NONE',  ( -25.98076211353311393, 53.43749999808803608, -3.000000000000132339 ) ) ;
#3814=CARTESIAN_POINT ( 'NONE',  ( -25.98076211353311393, 49.49999999999986500, -5.000000000000103029 ) ) ;
#3815=CARTESIAN_POINT ( 'NONE',  ( -25.17020516978313083, 51.41041666571061342, -6.403925809002825709 ) ) ;
#3821=AXIS2_PLACEMENT_3D ( 'NONE', #6130, #1858, #10357 ) ;
#3828=CARTESIAN_POINT ( 'NONE',  ( -26.79131905728310059, 49.95208333237728482, -6.403925809002825709 ) ) ;
#3833=CARTESIAN_POINT ( 'NONE',  ( -24.35964822603314772, 55.43541666571061199, -4.064049460664953983 ) ) ;
#3834=ORIENTED_EDGE ( 'NONE', *, *, #6155, .F. ) ;
#3841=( LENGTH_UNIT ( ) NAMED_UNIT ( * ) SI_UNIT ( .MILLI., .METRE. ) );
#3844=EDGE_CURVE ( 'NONE', #5854, #2292, #10358, .T. ) ;
#3854=CARTESIAN_POINT ( 'NONE',  ( -23.98076211353314235, 52.24166666666652503, -3.845299461620867554 ) ) ;
#3860=DIRECTION ( 'NONE',  ( 0.000000000000000000, 0.000000000000000000, 1.000000000000000000 ) ) ;
#3871=CARTESIAN_POINT ( 'NONE',  ( -24.98076211353312814, 51.71666666666652645, -6.732050807568954909 ) ) ;
#3872=CARTESIAN_POINT ( 'NONE',  ( -25.17020516978313083, 53.51041666571060773, -6.403925809002825709 ) ) ;
#3878=FACE_OUTER_BOUND ( 'NONE', #7752, .T. ) ;
#3882=CARTESIAN_POINT ( 'NONE',  ( -24.35964822603314772, 50.47708333237728340, -5.935950539335252074 ) ) ;
#3886=CARTESIAN_POINT ( 'NONE',  ( -25.98076211353311393, 53.08749999808803466, -7.000000000000072831 ) ) ;
#3892=ORIENTED_EDGE ( 'NONE', *, *, #4458, .T. ) ;
#3894=( LENGTH_UNIT ( ) NAMED_UNIT ( * ) SI_UNIT ( .MILLI., .METRE. ) );
#3899=CARTESIAN_POINT ( 'NONE',  ( -26.98076211353309972, 52.44583333142136894, -6.732050807568954909 ) ) ;
#3900=CARTESIAN_POINT ( 'NONE',  ( -27.98076211353308551, 53.40833333333319644, -3.845299461620869330 ) ) ;
#3901=CARTESIAN_POINT ( 'NONE',  ( -27.98076211353308551, 51.16249999808803750, -5.000000000000103029 ) ) ;
#3921=CARTESIAN_POINT ( 'NONE',  ( -25.98076211353311393, 49.89374999904395480, -6.871901078670400231 ) ) ;
#3923=CARTESIAN_POINT ( 'NONE',  ( -26.51666049839535688, 55.30626073911682994, -7.000000000000071942 ) ) ;
#3932=CARTESIAN_POINT ( 'NONE',  ( -27.60187600103308725, 52.92708333237727913, -4.064049460664955760 ) ) ;
#3936=EDGE_LOOP ( 'NONE', ( #10469, #8350, #7432, #128 ) ) ;
#3937=ORIENTED_EDGE ( 'NONE', *, *, #4069, .T. ) ;
#3947=CARTESIAN_POINT ( 'NONE',  ( -23.98076211353314235, 51.45416666475470180, -3.845299461620867554 ) ) ;
#3961=FACE_OUTER_BOUND ( 'NONE', #9048, .T. ) ;
#3968=CARTESIAN_POINT ( 'NONE',  ( -27.98076211353308551, 51.19166666666652787, -6.154700538379338504 ) ) ;
#3969=CARTESIAN_POINT ( 'NONE',  ( -25.17020516978313083, 50.30208333237728624, -3.596074190997380349 ) ) ;
#3976=DIRECTION ( 'NONE',  ( 0.000000000000000000, 1.000000000000000000, 0.000000000000000000 ) ) ;
#3979=CARTESIAN_POINT ( 'NONE',  ( -25.98076211353310683, 55.14374999904394059, -3.128098921329806714 ) ) ;
#3982=CARTESIAN_POINT ( 'NONE',  ( -25.98076211353311393, 50.02499999999986358, -2.690598923241634743 ) ) ;
#4000=CARTESIAN_POINT ( 'NONE',  ( -27.98076211353308551, 50.52083333142136468, -3.845299461620869330 ) ) ;
#4002=CARTESIAN_POINT ( 'NONE',  ( -27.98076211353308551, 53.29166666666652930, -6.154700538379338504 ) ) ;
#4003=DIRECTION ( 'NONE',  ( 0.000000000000000000, 0.000000000000000000, 1.000000000000000000 ) ) ;
#4004=B_SPLINE_CURVE_WITH_KNOTS ( 'NONE', 1,
 ( #10033, #4030 ),
 .UNSPECIFIED., .F., .F.,
 ( 2, 2 ),
 ( 0.000000000000000000, 1.000000000000000000 ),
 .UNSPECIFIED. ) ;
#4010=AXIS2_PLACEMENT_3D ( 'NONE', #4604, #5171, #6824 ) ;
#4011=CARTESIAN_POINT ( 'NONE',  ( -23.98076211353314235, 52.29999999999986215, -5.000000000000103029 ) ) ;
#4024=DIRECTION ( 'NONE',  ( 0.000000000000000000, 0.000000000000000000, 1.000000000000000000 ) ) ;
#4025=EDGE_CURVE ( 'NONE', #10232, #6011, #1627, .T. ) ;
#4027=CARTESIAN_POINT ( 'NONE',  ( -24.35964822603314417, 49.71874999904395054, -5.000000000000103029 ) ) ;
#4030=CARTESIAN_POINT ( 'NONE',  ( -24.35964822603314417, 49.71874999904395054, -5.000000000000103029 ) ) ;
#4035=CYLINDRICAL_SURFACE ( 'NONE', #4341, 1.999999999999971356 ) ;
#4039=CARTESIAN_POINT ( 'NONE',  ( -25.17020516978313083, 52.40208333237728766, -3.596074190997380349 ) ) ;
#4042=MECHANICAL_DESIGN_GEOMETRIC_PRESENTATION_REPRESENTATION('',(#10621),#5476);
#4044=CARTESIAN_POINT ( 'NONE',  ( -25.17020516978313083, 53.10208333237728340, -3.596074190997380349 ) ) ;
#4046=EDGE_CURVE ( 'NONE', #6011, #491, #4325, .T. ) ;
#4048=CARTESIAN_POINT ( 'NONE',  ( -26.79131905728310059, 55.72708333237728340, -6.403925809002825709 ) ) ;
#4054=CARTESIAN_POINT ( 'NONE',  ( -25.98076211353311038, 61.49999999999985789, -5.000000000000102141 ) ) ;
#4063=CARTESIAN_POINT ( 'NONE',  ( -24.98076211353312814, 50.22916666475470038, -6.732050807568954909 ) ) ;
#4069=EDGE_CURVE ( 'NONE', #4861, #8872, #10222, .T. ) ;
#4075=CARTESIAN_POINT ( 'NONE',  ( -25.44486372867087454, 51.36876073720500102, -3.000000000000132339 ) ) ;
#4086=CARTESIAN_POINT ( 'NONE',  ( -26.79131905728310059, 55.26041666571061484, -3.596074190997381237 ) ) ;
#4092=CARTESIAN_POINT ( 'NONE',  ( -24.35964822603314772, 51.23541666571061626, -4.064049460664953983 ) ) ;
#4093=CARTESIAN_POINT ( 'NONE',  ( -25.98076211353310683, 53.74374999904394912, -3.128098921329806714 ) ) ;
#4094=CIRCLE ( 'NONE', #2692, 1.999999999999971356 ) ;
#4096=CARTESIAN_POINT ( 'NONE',  ( -24.98076211353312814, 51.01666666666653072, -6.732050807568954909 ) ) ;
#4100=ORIENTED_EDGE ( 'NONE', *, *, #9474, .F. ) ;
#4106=VECTOR ( 'NONE', #5848, 1000.000000000000000 ) ;
#4113=CARTESIAN_POINT ( 'NONE',  ( -25.98076211353311393, 50.63749999808803182, -2.690598923241634743 ) ) ;
#4116=PRODUCT_DEFINITION_CONTEXT ( 'detailed design', #2307, 'design' ) ;
#4119=ORIENTED_EDGE ( 'NONE', *, *, #8713, .F. ) ;
#4124=DIRECTION ( 'NONE',  ( 0.000000000000000000, 1.000000000000000000, 0.000000000000000000 ) ) ;
#4133=( BOUNDED_CURVE ( )  B_SPLINE_CURVE ( 2, ( #5661, #642, #3199, #5707, #4991, #583, #8365, #2427, #7371, #3051, #8257, #7315, #9040, #10704, #6425, #10757, #6579, #9981, #9087, #1481, #5759, #9142, #1538, #4092, #9825, #4940, #8311, #694, #7480, #10868, #3257, #5816, #9201, #1593, #4143, #8991, #2210, #1382, #3489, #4267, #5216, #10263, #9372, #5104, #8421, #10152, #3433, #31, #88, #10205, #3316, #7710, #6871, #921, #6089, #2715, #1878, #2540, #6755, #2663, #1770, #6039, #5922, #9424, #9309, #5870, #6701, #10925, #2604, #5267, #8592, #1707, #9480, #5160, #7770, #10100, #7597, #2486, #6808, #10986, #8483, #3376, #6930, #866, #7655, #10320, #8542, #802, #8654, #1820, #5981, #9254, #4384, #4322, #1033, #978, #149, #3547, #4444, #1649, #5045, #4209, #2099, #1200, #2151 ),
 .UNSPECIFIED., .F., .F. ) 
 B_SPLINE_CURVE_WITH_KNOTS ( ( 3, 2, 2, 2, 2, 2, 2, 2, 2, 2, 2, 2, 2, 2, 2, 2, 2, 2, 2, 2, 2, 2, 2, 2, 2, 2, 2, 2, 2, 2, 2, 2, 2, 2, 2, 2, 2, 2, 2, 2, 2, 2, 2, 2, 2, 2, 2, 2, 2, 2, 2, 2, 3 ),
 ( 0.000000000000000000, 0.01944383300006776241, 0.03888766600013552482, 0.05833149900020328377, 0.07777533200027104965, 0.09721916500033880859, 0.1166629980004065675, 0.1361068310004743265, 0.1555506640005420993, 0.1749944970006098444, 0.1944383300006776172, 0.2138821630007453622, 0.2333259960008131351, 0.2527698290008809079, 0.2722136620009486530, 0.2916574950010164535, 0.3111013280010841986, 0.3305451610011519437, 0.3499889940012196887, 0.3694328270012874893, 0.3888766600013552344, 0.4083204930014230349, 0.4277643260014907245, 0.4472081590015585251, 0.4666519920016262701, 0.4860958250016940707, 0.5055396580017618158, 0.5249834910018296164, 0.5444273240018973059, 0.5638711570019651065, 0.5833149900020329071, 0.6027588230021005966, 0.6222026560021683972, 0.6416464890022361978, 0.6610903220023038873, 0.6805341550023716879, 0.6999779880024393774, 0.7194218210025072890, 0.7388656540025749786, 0.7583094870026426682, 0.7777533200027104687, 0.7971971530027782693, 0.8166409860028460699, 0.8360848190029137594, 0.8555286520029814490, 0.8749724850030493606, 0.8944163180031170501, 0.9138601510031848507, 0.9333039840032525403, 0.9527478170033203408, 0.9721916500033881414, 0.9916354830034558310, 1.000000000000000000 ),
 .UNSPECIFIED. ) 
 CURVE ( )  GEOMETRIC_REPRESENTATION_ITEM ( )  RATIONAL_B_SPLINE_CURVE ( ( 1.000000000000000000, 0.8660254037844387076, 1.000000000000000000, 0.8660254037844387076, 1.000000000000000000, 0.8660254037844387076, 1.000000000000000000, 0.8660254037844387076, 1.000000000000000000, 0.8660254037844387076, 1.000000000000000000, 0.8660254037844387076, 1.000000000000000000, 0.8660254037844387076, 1.000000000000000000, 0.8660254037844387076, 1.000000000000000000, 0.8660254037844387076, 1.000000000000000000, 0.8660254037844387076, 1.000000000000000000, 0.8660254037844387076, 1.000000000000000000, 0.8660254037844387076, 1.000000000000000000, 0.8660254037844387076, 1.000000000000000000, 0.8660254037844387076, 1.000000000000000000, 0.8660254037844387076, 1.000000000000000000, 0.8660254037844387076, 1.000000000000000000, 0.8660254037844387076, 1.000000000000000000, 0.8660254037844387076, 1.000000000000000000, 0.8660254037844387076, 1.000000000000000000, 0.8660254037844387076, 1.000000000000000000, 0.8660254037844387076, 1.000000000000000000, 0.8660254037844387076, 1.000000000000000000, 0.8660254037844387076, 1.000000000000000000, 0.8660254037844387076, 1.000000000000000000, 0.8660254037844387076, 1.000000000000000000, 0.8660254037844387076, 1.000000000000000000, 0.8660254037844387076, 1.000000000000000000, 0.8660254037844387076, 1.000000000000000000, 0.8660254037844387076, 1.000000000000000000, 0.8660254037844387076, 1.000000000000000000, 0.8660254037844387076, 1.000000000000000000, 0.8660254037844387076, 1.000000000000000000, 0.8660254037844387076, 1.000000000000000000, 0.8660254037844387076, 1.000000000000000000, 0.8660254037844387076, 1.000000000000000000, 0.8660254037844387076, 1.000000000000000000, 0.8660254037844387076, 1.000000000000000000, 0.8660254037844387076, 1.000000000000000000, 0.8660254037844387076, 1.000000000000000000, 0.8660254037844387076, 1.000000000000000000, 0.8660254037844387076, 1.000000000000000000, 0.8660254037844387076, 1.000000000000000000, 0.8660254037844387076, 1.000000000000000000, 0.8660254037844387076, 1.000000000000000000, 0.8660254037844387076, 1.000000000000000000, 0.8660254037844387076, 1.000000000000000000, 0.8660254037844387076, 1.000000000000000000, 0.8660254037844387076, 1.000000000000000000, 0.8660254037844387076, 1.000000000000000000, 0.8660254037844387076, 1.000000000000000000, 0.8660254037844387076, 1.000000000000000000, 0.9423656443075654199, 0.9343185842653825013 ) ) 
 REPRESENTATION_ITEM ( '' )  );
#4137=CARTESIAN_POINT ( 'NONE',  ( -25.17020516978313083, 51.00208333237728198, -3.596074190997380349 ) ) ;
#4143=CARTESIAN_POINT ( 'NONE',  ( -25.17020516978313083, 51.87708333237728198, -3.596074190997380349 ) ) ;
#4145=CARTESIAN_POINT ( 'NONE',  ( -24.35964822603314417, 54.61874999904395622, -5.000000000000103029 ) ) ;
#4147=CARTESIAN_POINT ( 'NONE',  ( -24.98076211353313170, 50.78333333333319644, -3.267949192431250705 ) ) ;
#4161=AXIS2_PLACEMENT_3D ( 'NONE', #5553, #8933, #4725 ) ;
#4167=CARTESIAN_POINT ( 'NONE',  ( -23.98076211353314235, 54.25416666475469896, -3.845299461620867554 ) ) ;
#4172=CARTESIAN_POINT ( 'NONE',  ( -26.51666049839534622, 50.31876073720500386, -7.000000000000073719 ) ) ;
#4178=ORIENTED_EDGE ( 'NONE', *, *, #6072, .F. ) ;
#4195=CARTESIAN_POINT ( 'NONE',  ( -26.51666049839535688, 54.51876073720499249, -7.000000000000071942 ) ) ;
#4199=CARTESIAN_POINT ( 'NONE',  ( -27.60187600103308014, 52.92708333237728624, -4.064049460664955760 ) ) ;
#4208=( BOUNDED_SURFACE ( )  B_SPLINE_SURFACE ( 1, 2, ( 
 ( #8277, #4844, #4063, #8172, #8218, #2289, #6553, #4000, #3170, #4113, #662, #7280, #548, #3066, #5626, #1347, #8121, #7445, #9105, #3020, #9842, #7332, #1558, #3947, #10780, #1451, #9951, #6441, #10836, #503, #7389, #2335, #1501, #604, #5728, #3222, #6395, #4746, #4903, #2234, #3899, #9787, #2177, #6600, #10628, #4796, #10000, #5572, #2387, #10675, #5778, #8952, #9011, #9162, #1403, #10720, #4962, #3119, #6496, #9898, #8332, #5678, #9056, #711, #9442, #1788, #5890, #10285, #9336, #4344, #3278, #4167, #10061, #5177, #6724, #10174, #1614, #7560, #3509, #9276, #10946, #6899, #5126, #5012, #6054, #4286, #10117, #6661, #941, #8505, #2679, #885, #827, #8388, #2451, #3338, #2563, #4231, #2504, #7676, #1838, #764, #5838, #7501, #1669 ),
 ( #52, #5068, #8448, #9221, #3455, #8558, #5946, #7620, #2626, #10887, #5231, #6835, #10228, #6004, #1730, #9390, #7731, #111, #3678, #996, #3394, #6776, #8617, #273, #2120, #1161, #10391, #10336, #8675, #4565, #5507, #8775, #2899, #2790, #7951, #9500, #2848, #7161, #2059, #6105, #9557, #8890, #2731, #1957, #5391, #6219, #10454, #1105, #5338, #3564, #4461, #9604, #4509, #3613, #329, #9721, #1900, #5286, #4405, #1050, #6946, #2004, #8006, #7792, #3780, #8724, #3724, #1225, #168, #7842, #7062, #5449, #6166, #7112, #10508, #214, #7001, #7895, #6269, #3670, #9664, #8838, #4621, #378, #10558, #2954, #6328, #4730, #8264, #2321, #648, #9937, #4673, #5714, #3206, #3833, #9092, #1486, #8997, #2371, #4048, #9045, #6539, #4833, #8108 ) ),
 .UNSPECIFIED., .F., .F., .F. ) 
 B_SPLINE_SURFACE_WITH_KNOTS ( ( 2, 2 ),
 ( 3, 2, 2, 2, 2, 2, 2, 2, 2, 2, 2, 2, 2, 2, 2, 2, 2, 2, 2, 2, 2, 2, 2, 2, 2, 2, 2, 2, 2, 2, 2, 2, 2, 2, 2, 2, 2, 2, 2, 2, 2, 2, 2, 2, 2, 2, 2, 2, 2, 2, 2, 2, 3 ),
 ( 0.000000000000000000, 1.000000000000000000 ),
 ( 0.000000000000000000, 0.01851851851851851749, 0.03703703703703703498, 0.05555555555555555247, 0.07407407407407406996, 0.09259259259259258745, 0.1111111111111111049, 0.1296296296296296224, 0.1481481481481481399, 0.1666666666666666574, 0.1851851851851851749, 0.2037037037037036924, 0.2222222222222222099, 0.2407407407407407274, 0.2592592592592592449, 0.2777777777777777901, 0.2962962962962962798, 0.3148148148148148251, 0.3333333333333333148, 0.3518518518518518601, 0.3703703703703703498, 0.3888888888888888951, 0.4074074074074073848, 0.4259259259259259300, 0.4444444444444444198, 0.4629629629629629650, 0.4814814814814814548, 0.5000000000000000000, 0.5185185185185184897, 0.5370370370370370905, 0.5555555555555555802, 0.5740740740740740700, 0.5925925925925925597, 0.6111111111111111605, 0.6296296296296296502, 0.6481481481481481399, 0.6666666666666666297, 0.6851851851851852304, 0.7037037037037037202, 0.7222222222222222099, 0.7407407407407406996, 0.7592592592592593004, 0.7777777777777777901, 0.7962962962962962798, 0.8148148148148147696, 0.8333333333333333703, 0.8518518518518518601, 0.8703703703703703498, 0.8888888888888888395, 0.9074074074074074403, 0.9259259259259259300, 0.9444444444444444198, 0.9524109016187282117 ),
 .UNSPECIFIED. ) 
 GEOMETRIC_REPRESENTATION_ITEM ( )  RATIONAL_B_SPLINE_SURFACE ( (
 ( 1.000000000000000000, 0.8660254037844387076, 1.000000000000000000, 0.8660254037844387076, 1.000000000000000000, 0.8660254037844387076, 1.000000000000000000, 0.8660254037844387076, 1.000000000000000000, 0.8660254037844387076, 1.000000000000000000, 0.8660254037844387076, 1.000000000000000000, 0.8660254037844387076, 1.000000000000000000, 0.8660254037844387076, 1.000000000000000000, 0.8660254037844387076, 1.000000000000000000, 0.8660254037844387076, 1.000000000000000000, 0.8660254037844387076, 1.000000000000000000, 0.8660254037844387076, 1.000000000000000000, 0.8660254037844387076, 1.000000000000000000, 0.8660254037844387076, 1.000000000000000000, 0.8660254037844387076, 1.000000000000000000, 0.8660254037844387076, 1.000000000000000000, 0.8660254037844387076, 1.000000000000000000, 0.8660254037844387076, 1.000000000000000000, 0.8660254037844387076, 1.000000000000000000, 0.8660254037844387076, 1.000000000000000000, 0.8660254037844387076, 1.000000000000000000, 0.8660254037844387076, 1.000000000000000000, 0.8660254037844387076, 1.000000000000000000, 0.8660254037844387076, 1.000000000000000000, 0.8660254037844387076, 1.000000000000000000, 0.8660254037844387076, 1.000000000000000000, 0.8660254037844387076, 1.000000000000000000, 0.8660254037844387076, 1.000000000000000000, 0.8660254037844387076, 1.000000000000000000, 0.8660254037844387076, 1.000000000000000000, 0.8660254037844387076, 1.000000000000000000, 0.8660254037844387076, 1.000000000000000000, 0.8660254037844387076, 1.000000000000000000, 0.8660254037844387076, 1.000000000000000000, 0.8660254037844387076, 1.000000000000000000, 0.8660254037844387076, 1.000000000000000000, 0.8660254037844387076, 1.000000000000000000, 0.8660254037844387076, 1.000000000000000000, 0.8660254037844387076, 1.000000000000000000, 0.8660254037844387076, 1.000000000000000000, 0.8660254037844387076, 1.000000000000000000, 0.8660254037844387076, 1.000000000000000000, 0.8660254037844387076, 1.000000000000000000, 0.8660254037844387076, 1.000000000000000000, 0.8660254037844387076, 1.000000000000000000, 0.8660254037844387076, 1.000000000000000000, 0.8660254037844387076, 1.000000000000000000, 0.8660254037844387076, 1.000000000000000000, 0.8660254037844387076, 1.000000000000000000, 0.8660254037844387076, 1.000000000000000000, 0.8660254037844387076, 1.000000000000000000, 0.9423656443075654199, 0.9343185842653825013),
 ( 1.000000000000000000, 0.8660254037844387076, 1.000000000000000000, 0.8660254037844387076, 1.000000000000000000, 0.8660254037844387076, 1.000000000000000000, 0.8660254037844387076, 1.000000000000000000, 0.8660254037844387076, 1.000000000000000000, 0.8660254037844387076, 1.000000000000000000, 0.8660254037844387076, 1.000000000000000000, 0.8660254037844387076, 1.000000000000000000, 0.8660254037844387076, 1.000000000000000000, 0.8660254037844387076, 1.000000000000000000, 0.8660254037844387076, 1.000000000000000000, 0.8660254037844387076, 1.000000000000000000, 0.8660254037844387076, 1.000000000000000000, 0.8660254037844387076, 1.000000000000000000, 0.8660254037844387076, 1.000000000000000000, 0.8660254037844387076, 1.000000000000000000, 0.8660254037844387076, 1.000000000000000000, 0.8660254037844387076, 1.000000000000000000, 0.8660254037844387076, 1.000000000000000000, 0.8660254037844387076, 1.000000000000000000, 0.8660254037844387076, 1.000000000000000000, 0.8660254037844387076, 1.000000000000000000, 0.8660254037844387076, 1.000000000000000000, 0.8660254037844387076, 1.000000000000000000, 0.8660254037844387076, 1.000000000000000000, 0.8660254037844387076, 1.000000000000000000, 0.8660254037844387076, 1.000000000000000000, 0.8660254037844387076, 1.000000000000000000, 0.8660254037844387076, 1.000000000000000000, 0.8660254037844387076, 1.000000000000000000, 0.8660254037844387076, 1.000000000000000000, 0.8660254037844387076, 1.000000000000000000, 0.8660254037844387076, 1.000000000000000000, 0.8660254037844387076, 1.000000000000000000, 0.8660254037844387076, 1.000000000000000000, 0.8660254037844387076, 1.000000000000000000, 0.8660254037844387076, 1.000000000000000000, 0.8660254037844387076, 1.000000000000000000, 0.8660254037844387076, 1.000000000000000000, 0.8660254037844387076, 1.000000000000000000, 0.8660254037844387076, 1.000000000000000000, 0.8660254037844387076, 1.000000000000000000, 0.8660254037844387076, 1.000000000000000000, 0.8660254037844387076, 1.000000000000000000, 0.8660254037844387076, 1.000000000000000000, 0.8660254037844387076, 1.000000000000000000, 0.8660254037844387076, 1.000000000000000000, 0.8660254037844387076, 1.000000000000000000, 0.8660254037844387076, 1.000000000000000000, 0.8660254037844387076, 1.000000000000000000, 0.8660254037844387076, 1.000000000000000000, 0.9423656443075654199, 0.9343185842653825013) ) ) 
 REPRESENTATION_ITEM ( '' )  SURFACE ( )  );
#4209=CARTESIAN_POINT ( 'NONE',  ( -27.60187600103308725, 55.78541666571062052, -5.935950539335252074 ) ) ;
#4213=CIRCLE ( 'NONE', #2096, 1.999999999999971356 ) ;
#4214=CARTESIAN_POINT ( 'NONE',  ( -27.98076211353308551, 51.94999999999986784, -5.000000000000103029 ) ) ;
#4215=ORIENTED_EDGE ( 'NONE', *, *, #8444, .F. ) ;
#4217=ORIENTED_EDGE ( 'NONE', *, *, #10142, .T. ) ;
#4231=CARTESIAN_POINT ( 'NONE',  ( -23.98076211353314235, 55.77083333142137178, -6.154700538379337615 ) ) ;
#4234=CARTESIAN_POINT ( 'NONE',  ( -23.98076211353314235, 53.64166666666653072, -3.845299461620867554 ) ) ;
#4236=CARTESIAN_POINT ( 'NONE',  ( -25.00795256721317372, 58.26617124284993565, -3.251596195468438033 ) ) ;
#4243=EDGE_CURVE ( 'NONE', #491, #6512, #8438, .T. ) ;
#4244=CARTESIAN_POINT ( 'NONE',  ( -25.98076211353310683, 53.52499999999986358, -3.000000000000132339 ) ) ;
#4254=ADVANCED_FACE ( 'NONE', ( #10136 ), #5089, .T. ) ;
#4255=DIRECTION ( 'NONE',  ( 0.000000000000000000, 1.000000000000000000, 0.000000000000000000 ) ) ;
#4256=CARTESIAN_POINT ( 'NONE',  ( -25.98076211353311393, 54.48749999808803324, -7.000000000000072831 ) ) ;
#4260=CARTESIAN_POINT ( 'NONE',  ( -24.35964822603314417, 53.21874999904395764, -5.000000000000103029 ) ) ;
#4261=CARTESIAN_POINT ( 'NONE',  ( -24.35964822603314417, 49.89374999904394770, -5.000000000000103029 ) ) ;
#4267=CARTESIAN_POINT ( 'NONE',  ( -25.98076211353310683, 52.16874999904395338, -6.871901078670399343 ) ) ;
#4268=CARTESIAN_POINT ( 'NONE',  ( -23.98076211353314235, 50.84166666666652645, -3.845299461620867554 ) ) ;
#4271=CARTESIAN_POINT ( 'NONE',  ( -25.98076211353311393, 51.77499999999986358, -7.309401076758571314 ) ) ;
#4273=( BOUNDED_CURVE ( )  B_SPLINE_CURVE ( 2, ( #3813, #7254, #6372, #9760, #2152, #1311, #8707, #1086, #2880 ),
 .UNSPECIFIED., .F., .F. ) 
 B_SPLINE_CURVE_WITH_KNOTS ( ( 3, 2, 2, 2, 3 ),
 ( 0.5277777777777777901, 0.5370370370370370905, 0.5555555555555555802, 0.5740740740740740700, 0.5833333333333333703 ),
 .UNSPECIFIED. ) 
 CURVE ( )  GEOMETRIC_REPRESENTATION_ITEM ( )  RATIONAL_B_SPLINE_CURVE ( ( 0.9330127018922194093, 0.9330127018922194093, 1.000000000000000000, 0.8660254037844387076, 1.000000000000000000, 0.8660254037844387076, 1.000000000000000000, 0.9330127018922189652, 0.9330127018922194093 ) ) 
 REPRESENTATION_ITEM ( '' )  );
#4274=VERTEX_POINT ( 'NONE', #294 ) ;
#4282=FACE_OUTER_BOUND ( 'NONE', #9828, .T. ) ;
#4286=CARTESIAN_POINT ( 'NONE',  ( -23.98076211353314235, 55.07083333142136894, -6.154700538379337615 ) ) ;
#4292=ORIENTED_EDGE ( 'NONE', *, *, #7162, .F. ) ;
#4296=DIRECTION ( 'NONE',  ( 0.000000000000000000, 0.000000000000000000, 1.000000000000000000 ) ) ;
#4297=CARTESIAN_POINT ( 'NONE',  ( -25.47290043343602051, 58.87139657625925082, -6.938381116177147589 ) ) ;
#4299=CARTESIAN_POINT ( 'NONE',  ( -27.60187600103308014, 52.81041666571061199, -5.935950539335252074 ) ) ;
#4303=CARTESIAN_POINT ( 'NONE',  ( -26.94773701350929329, 58.26330508548400644, -6.750767313052078222 ) ) ;
#4307=CARTESIAN_POINT ( 'NONE',  ( -26.51666049839534622, 51.80626073911682283, -7.000000000000073719 ) ) ;
#4310=VECTOR ( 'NONE', #10750, 1000.000000000000000 ) ;
#4311=CARTESIAN_POINT ( 'NONE',  ( -23.98076211353314235, 55.77083333142137178, -6.154700538379337615 ) ) ;
#4314=CARTESIAN_POINT ( 'NONE',  ( -24.35964822603314772, 55.26041666571062194, -4.064049460664953983 ) ) ;
#4315=ADVANCED_FACE ( 'NONE', ( #2753 ), #10413, .T. ) ;
#4322=CARTESIAN_POINT ( 'NONE',  ( -25.98076211353310683, 55.31874999904394485, -3.128098921329806714 ) ) ;
#4323=CARTESIAN_POINT ( 'NONE',  ( -25.44486372867087454, 51.04373926088290858, -7.000000000000073719 ) ) ;
#4325=( BOUNDED_CURVE ( )  B_SPLINE_CURVE ( 2, ( #8924, #1312, #8147, #469, #2257, #8039, #3871, #3041, #6415 ),
 .UNSPECIFIED., .F., .F. ) 
 B_SPLINE_CURVE_WITH_KNOTS ( ( 3, 2, 2, 2, 3 ),
 ( 0.3055555555555555802, 0.3148148148148148251, 0.3333333333333333148, 0.3518518518518518601, 0.3611111111111111049 ),
 .UNSPECIFIED. ) 
 CURVE ( )  GEOMETRIC_REPRESENTATION_ITEM ( )  RATIONAL_B_SPLINE_CURVE ( ( 0.9330127018922194093, 0.9330127018922195203, 1.000000000000000000, 0.8660254037844387076, 1.000000000000000000, 0.8660254037844387076, 1.000000000000000000, 0.9330127018922194093, 0.9330127018922194093 ) ) 
 REPRESENTATION_ITEM ( '' )  );
#4327=CARTESIAN_POINT ( 'NONE',  ( -26.98076211353309972, 51.13333333333319786, -6.732050807568954909 ) ) ;
#4337=CARTESIAN_POINT ( 'NONE',  ( -26.51666049839535333, 52.00623925897107114, -3.000000000000132339 ) ) ;
#4341=AXIS2_PLACEMENT_3D ( 'NONE', #3147, #6529, #9928 ) ;
#4344=CARTESIAN_POINT ( 'NONE',  ( -25.98076211353311393, 54.13749999808803182, -2.690598923241634743 ) ) ;
#4345=CARTESIAN_POINT ( 'NONE',  ( -23.98076211353314235, 53.75833333333319786, -6.154700538379337615 ) ) ;
#4356=CARTESIAN_POINT ( 'NONE',  ( -25.17020516978313083, 50.53541666571062052, -6.403925809002825709 ) ) ;
#4371=CARTESIAN_POINT ( 'NONE',  ( -27.98076211353308551, 52.59166666666651935, -6.154700538379338504 ) ) ;
#4373=CARTESIAN_POINT ( 'NONE',  ( -27.60187600103308014, 54.32708333237728482, -4.064049460664955760 ) ) ;
#4384=CARTESIAN_POINT ( 'NONE',  ( -26.79131905728310059, 55.26041666571061484, -3.596074190997381237 ) ) ;
#4397=LINE ( 'NONE', #819, #9672 ) ;
#4405=CARTESIAN_POINT ( 'NONE',  ( -25.17020516978313083, 53.27708333237728056, -3.596074190997380349 ) ) ;
#4419=( GEOMETRIC_REPRESENTATION_CONTEXT ( 3 ) GLOBAL_UNCERTAINTY_ASSIGNED_CONTEXT ( ( #5322 ) ) GLOBAL_UNIT_ASSIGNED_CONTEXT ( ( #3894, #9008, #3679 ) ) REPRESENTATION_CONTEXT ( 'NONE', 'WORKASPACE' ) );
#4420=CARTESIAN_POINT ( 'NONE',  ( -27.60187600103308014, 52.11041666571061626, -5.935950539335252074 ) ) ;
#4433=CARTESIAN_POINT ( 'NONE',  ( -25.98076211353311393, 52.47499999999985931, -7.000000000000072831 ) ) ;
#4435=CARTESIAN_POINT ( 'NONE',  ( -25.17020516978313083, 55.20208333237728482, -3.596074190997380349 ) ) ;
#4444=CARTESIAN_POINT ( 'NONE',  ( -25.17020516978313083, 55.61041666571061626, -6.403925809002825709 ) ) ;
#4445=CARTESIAN_POINT ( 'NONE',  ( -23.98076211353314235, 55.04166666666652930, -3.845299461620867554 ) ) ;
#4447=CARTESIAN_POINT ( 'NONE',  ( -23.98076211353314235, 54.34166666666652645, -3.845299461620867554 ) ) ;
#4451=CARTESIAN_POINT ( 'NONE',  ( -23.98076211353314235, 50.75416666475469896, -3.845299461620867554 ) ) ;
#4456=CARTESIAN_POINT ( 'NONE',  ( -25.98076211353311393, 54.57499999999986073, -7.000000000000072831 ) ) ;
#4458=EDGE_CURVE ( 'NONE', #5004, #5575, #2606, .T. ) ;
#4461=CARTESIAN_POINT ( 'NONE',  ( -25.17020516978313083, 52.81041666571061199, -6.403925809002825709 ) ) ;
#4484=PLANE ( 'NONE',  #4822 ) ;
#4485=CARTESIAN_POINT ( 'NONE',  ( -25.98076211353311393, 50.63749999808803892, -3.000000000000132339 ) ) ;
#4497=CARTESIAN_POINT ( 'NONE',  ( -24.98076211353312814, 55.21666666666653356, -6.732050807568954909 ) ) ;
#4502=CARTESIAN_POINT ( 'NONE',  ( -25.98076211353311393, 49.49999999999986500, -5.000000000000103029 ) ) ;
#4505=CARTESIAN_POINT ( 'NONE',  ( -27.98076211353308551, 51.92083333142137036, -3.845299461620869330 ) ) ;
#4508=CARTESIAN_POINT ( 'NONE',  ( -24.17020516978314504, 49.60937499952190421, -5.000000000000103029 ) ) ;
#4509=CARTESIAN_POINT ( 'NONE',  ( -26.79131905728310059, 52.92708333237727913, -6.403925809002825709 ) ) ;
#4512=CARTESIAN_POINT ( 'NONE',  ( -25.98076211353311393, 50.98749999808804034, -7.000000000000073719 ) ) ;
#4521=CARTESIAN_POINT ( 'NONE',  ( -24.35964822603314417, 53.91874999904395338, -5.000000000000103029 ) ) ;
#4530=CARTESIAN_POINT ( 'NONE',  ( -25.98076211353311393, 54.22499999999985931, -3.000000000000132339 ) ) ;
#4532=CARTESIAN_POINT ( 'NONE',  ( -26.51666049839535688, 52.41876073720499818, -7.000000000000071942 ) ) ;
#4537=( LENGTH_UNIT ( ) NAMED_UNIT ( * ) SI_UNIT ( .MILLI., .METRE. ) );
#4548=ADVANCED_FACE ( 'NONE', ( #2305 ), #10743, .T. ) ;
#4551=CARTESIAN_POINT ( 'NONE',  ( -25.98076211353311393, 53.91874999904394627, -3.128098921329806714 ) ) ;
#4553=CARTESIAN_POINT ( 'NONE',  ( -27.98076211353308551, 55.44999999999986073, -5.000000000000103029 ) ) ;
#4555=EDGE_LOOP ( 'NONE', ( #5712, #1675, #7667 ) ) ;
#4562=DIRECTION ( 'NONE',  ( 0.000000000000000000, -0.7071067811865420216, -0.7071067811865531239 ) ) ;
#4565=CARTESIAN_POINT ( 'NONE',  ( -27.60187600103308014, 51.58541666571061768, -5.935950539335252074 ) ) ;
#4566=VERTEX_POINT ( 'NONE', #6515 ) ;
#4568=ORIENTED_EDGE ( 'NONE', *, *, #3686, .F. ) ;
#4573=( BOUNDED_SURFACE ( )  B_SPLINE_SURFACE ( 1, 2, ( 
 ( #9997, #9272, #47, #3451, #1666, #10883, #6830, #5065, #8443, #822, #10225, #3275, #7728, #6658, #106, #10652, #7991, #4769, #8148, #8040, #1989, #4608, #5544, #5435, #1313, #2833, #3815, #9706, #2102, #4712, #6254, #5495, #7203, #7148, #2041, #9763, #6315, #8759, #10279, #1204, #8879, #10598, #10542, #1264, #9647, #2938, #8822, #4658, #413, #6374, #3709, #8981, #362, #3765, #2199, #2995, #2153, #6204, #8925, #8093, #470, #5375, #3872, #7256, #3042, #6416, #9814, #5595, #1142, #4551, #1371, #523, #6893, #9588, #7935, #313, #10491, #7099, #2882, #5863, #9191, #10807, #1642, #687, #9923, #7470, #9245, #10031, #4869, #8303, #2420, #2310, #4086, #9034, #2359, #6693, #1585, #8248, #10860, #3250, #4983, #9079, #4931, #5749, #9974 ),
 ( #4027, #10748, #6624, #3921, #3192, #5805, #8357, #7360, #8412, #736, #3969, #634, #5701, #7415, #7306, #6573, #6468, #9134, #7527, #1530, #5037, #10698, #4137, #9869, #1475, #10917, #3309, #10090, #3091, #2479, #2258, #5652, #1425, #3140, #4818, #8196, #574, #6520, #10196, #6921, #2758, #9527, #10362, #6862, #5153, #9414, #1927, #859, #6801, #6134, #6081, #8475, #1698, #5314, #795, #4199, #10255, #8534, #1812, #7589, #4260, #2595, #10979, #9470, #7645, #5095, #5206, #3367, #9364, #3539, #2655, #7758, #22, #1023, #3424, #8583, #966, #2705, #6030, #4373, #1863, #6747, #2531, #139, #5974, #5916, #9299, #3482, #10310, #1762, #911, #5259, #10144, #8642, #4435, #4314, #7701, #7817, #189, #77, #3590, #6974, #8747, #10530, #1129 ) ),
 .UNSPECIFIED., .F., .F., .T. ) 
 B_SPLINE_SURFACE_WITH_KNOTS ( ( 2, 2 ),
 ( 3, 2, 2, 2, 2, 2, 2, 2, 2, 2, 2, 2, 2, 2, 2, 2, 2, 2, 2, 2, 2, 2, 2, 2, 2, 2, 2, 2, 2, 2, 2, 2, 2, 2, 2, 2, 2, 2, 2, 2, 2, 2, 2, 2, 2, 2, 2, 2, 2, 2, 2, 2, 3 ),
 ( 0.000000000000000000, 1.000000000000000000 ),
 ( 0.000000000000000000, 0.01851851851851851749, 0.03703703703703703498, 0.05555555555555555247, 0.07407407407407406996, 0.09259259259259258745, 0.1111111111111111049, 0.1296296296296296224, 0.1481481481481481399, 0.1666666666666666574, 0.1851851851851851749, 0.2037037037037036924, 0.2222222222222222099, 0.2407407407407407274, 0.2592592592592592449, 0.2777777777777777901, 0.2962962962962962798, 0.3148148148148148251, 0.3333333333333333148, 0.3518518518518518601, 0.3703703703703703498, 0.3888888888888888951, 0.4074074074074073848, 0.4259259259259259300, 0.4444444444444444198, 0.4629629629629629650, 0.4814814814814814548, 0.5000000000000000000, 0.5185185185185184897, 0.5370370370370370905, 0.5555555555555555802, 0.5740740740740740700, 0.5925925925925925597, 0.6111111111111111605, 0.6296296296296296502, 0.6481481481481481399, 0.6666666666666666297, 0.6851851851851852304, 0.7037037037037037202, 0.7222222222222222099, 0.7407407407407406996, 0.7592592592592593004, 0.7777777777777777901, 0.7962962962962962798, 0.8148148148148147696, 0.8333333333333333703, 0.8518518518518518601, 0.8703703703703703498, 0.8888888888888888395, 0.9074074074074074403, 0.9259259259259259300, 0.9444444444444444198, 0.9524110019551522699 ),
 .UNSPECIFIED. ) 
 GEOMETRIC_REPRESENTATION_ITEM ( )  RATIONAL_B_SPLINE_SURFACE ( (
 ( 1.000000000000000000, 0.8660254037844387076, 1.000000000000000000, 0.8660254037844387076, 1.000000000000000000, 0.8660254037844387076, 1.000000000000000000, 0.8660254037844387076, 1.000000000000000000, 0.8660254037844387076, 1.000000000000000000, 0.8660254037844387076, 1.000000000000000000, 0.8660254037844387076, 1.000000000000000000, 0.8660254037844387076, 1.000000000000000000, 0.8660254037844387076, 1.000000000000000000, 0.8660254037844387076, 1.000000000000000000, 0.8660254037844387076, 1.000000000000000000, 0.8660254037844387076, 1.000000000000000000, 0.8660254037844387076, 1.000000000000000000, 0.8660254037844387076, 1.000000000000000000, 0.8660254037844387076, 1.000000000000000000, 0.8660254037844387076, 1.000000000000000000, 0.8660254037844387076, 1.000000000000000000, 0.8660254037844387076, 1.000000000000000000, 0.8660254037844387076, 1.000000000000000000, 0.8660254037844387076, 1.000000000000000000, 0.8660254037844387076, 1.000000000000000000, 0.8660254037844387076, 1.000000000000000000, 0.8660254037844387076, 1.000000000000000000, 0.8660254037844387076, 1.000000000000000000, 0.8660254037844387076, 1.000000000000000000, 0.8660254037844387076, 1.000000000000000000, 0.8660254037844387076, 1.000000000000000000, 0.8660254037844387076, 1.000000000000000000, 0.8660254037844387076, 1.000000000000000000, 0.8660254037844387076, 1.000000000000000000, 0.8660254037844387076, 1.000000000000000000, 0.8660254037844387076, 1.000000000000000000, 0.8660254037844387076, 1.000000000000000000, 0.8660254037844387076, 1.000000000000000000, 0.8660254037844387076, 1.000000000000000000, 0.8660254037844387076, 1.000000000000000000, 0.8660254037844387076, 1.000000000000000000, 0.8660254037844387076, 1.000000000000000000, 0.8660254037844387076, 1.000000000000000000, 0.8660254037844387076, 1.000000000000000000, 0.8660254037844387076, 1.000000000000000000, 0.8660254037844387076, 1.000000000000000000, 0.8660254037844387076, 1.000000000000000000, 0.8660254037844387076, 1.000000000000000000, 0.8660254037844387076, 1.000000000000000000, 0.8660254037844387076, 1.000000000000000000, 0.8660254037844387076, 1.000000000000000000, 0.8660254037844387076, 1.000000000000000000, 0.8660254037844387076, 1.000000000000000000, 0.8660254037844387076, 1.000000000000000000, 0.8660254037844387076, 1.000000000000000000, 0.9423649184108428001, 0.9343183815700366601),
 ( 1.000000000000000000, 0.8660254037844387076, 1.000000000000000000, 0.8660254037844387076, 1.000000000000000000, 0.8660254037844387076, 1.000000000000000000, 0.8660254037844387076, 1.000000000000000000, 0.8660254037844387076, 1.000000000000000000, 0.8660254037844387076, 1.000000000000000000, 0.8660254037844387076, 1.000000000000000000, 0.8660254037844387076, 1.000000000000000000, 0.8660254037844387076, 1.000000000000000000, 0.8660254037844387076, 1.000000000000000000, 0.8660254037844387076, 1.000000000000000000, 0.8660254037844387076, 1.000000000000000000, 0.8660254037844387076, 1.000000000000000000, 0.8660254037844387076, 1.000000000000000000, 0.8660254037844387076, 1.000000000000000000, 0.8660254037844387076, 1.000000000000000000, 0.8660254037844387076, 1.000000000000000000, 0.8660254037844387076, 1.000000000000000000, 0.8660254037844387076, 1.000000000000000000, 0.8660254037844387076, 1.000000000000000000, 0.8660254037844387076, 1.000000000000000000, 0.8660254037844387076, 1.000000000000000000, 0.8660254037844387076, 1.000000000000000000, 0.8660254037844387076, 1.000000000000000000, 0.8660254037844387076, 1.000000000000000000, 0.8660254037844387076, 1.000000000000000000, 0.8660254037844387076, 1.000000000000000000, 0.8660254037844387076, 1.000000000000000000, 0.8660254037844387076, 1.000000000000000000, 0.8660254037844387076, 1.000000000000000000, 0.8660254037844387076, 1.000000000000000000, 0.8660254037844387076, 1.000000000000000000, 0.8660254037844387076, 1.000000000000000000, 0.8660254037844387076, 1.000000000000000000, 0.8660254037844387076, 1.000000000000000000, 0.8660254037844387076, 1.000000000000000000, 0.8660254037844387076, 1.000000000000000000, 0.8660254037844387076, 1.000000000000000000, 0.8660254037844387076, 1.000000000000000000, 0.8660254037844387076, 1.000000000000000000, 0.8660254037844387076, 1.000000000000000000, 0.8660254037844387076, 1.000000000000000000, 0.8660254037844387076, 1.000000000000000000, 0.8660254037844387076, 1.000000000000000000, 0.8660254037844387076, 1.000000000000000000, 0.8660254037844387076, 1.000000000000000000, 0.8660254037844387076, 1.000000000000000000, 0.8660254037844387076, 1.000000000000000000, 0.8660254037844387076, 1.000000000000000000, 0.8660254037844387076, 1.000000000000000000, 0.8660254037844387076, 1.000000000000000000, 0.9423649184108428001, 0.9343183815700366601) ) ) 
 REPRESENTATION_ITEM ( '' )  SURFACE ( )  );
#4576=CARTESIAN_POINT ( 'NONE',  ( -25.98076211353311393, 55.49374999904395622, -6.871901078670400231 ) ) ;
#4587=CARTESIAN_POINT ( 'NONE',  ( -23.98076211353314235, 50.14166666666653072, -3.845299461620867554 ) ) ;
#4591=CARTESIAN_POINT ( 'NONE',  ( -25.98076211353311393, 52.38749999808802471, -7.000000000000072831 ) ) ;
#4604=CARTESIAN_POINT ( 'NONE',  ( -25.98076211353311038, 60.99999999999985789, -5.000000000000102141 ) ) ;
#4605=CARTESIAN_POINT ( 'NONE',  ( -24.98076211353312814, 55.12916666475470606, -6.732050807568954909 ) ) ;
#4608=CARTESIAN_POINT ( 'NONE',  ( -25.98076211353311393, 51.11874999904394201, -3.128098921329806714 ) ) ;
#4614=CYLINDRICAL_SURFACE ( 'NONE', #2751, 1.999999999999971356 ) ;
#4617=DIRECTION ( 'NONE',  ( 0.000000000000000000, 1.000000000000000000, 0.000000000000000000 ) ) ;
#4618=CARTESIAN_POINT ( 'NONE',  ( -27.60187600103308725, 50.12708333237728198, -4.064049460664955760 ) ) ;
#4621=CARTESIAN_POINT ( 'NONE',  ( -25.17020516978313083, 54.67708333237727913, -3.596074190997380349 ) ) ;
#4629=FILL_AREA_STYLE_COLOUR ( '', #1208 ) ;
#4632=CARTESIAN_POINT ( 'NONE',  ( -25.98076211353311393, 54.09374999904395054, -6.871901078670400231 ) ) ;
#4639=CARTESIAN_POINT ( 'NONE',  ( -25.98076211353311393, 50.37499999999987210, -7.000000000000073719 ) ) ;
#4640=CARTESIAN_POINT ( 'NONE',  ( -26.59846429743006269, 58.79685839844216133, -3.095304781643430925 ) ) ;
#4643=CARTESIAN_POINT ( 'NONE',  ( -25.98076211353311038, 49.67499999999986215, -7.000000000000072831 ) ) ;
#4658=CARTESIAN_POINT ( 'NONE',  ( -24.35964822603314772, 52.63541666571061484, -4.064049460664953983 ) ) ;
#4660=CARTESIAN_POINT ( 'NONE',  ( -27.98076211353308196, 55.47306177707831409, -4.543495204426306167 ) ) ;
#4666=CARTESIAN_POINT ( 'NONE',  ( -27.78269821382355431, 55.90794815475196344, -4.132229125461595487 ) ) ;
#4668=CARTESIAN_POINT ( 'NONE',  ( -25.17020516978313083, 49.83541666571061768, -6.403925809002825709 ) ) ;
#4673=CARTESIAN_POINT ( 'NONE',  ( -26.79131905728310059, 55.26041666571061484, -3.596074190997381237 ) ) ;
#4683=EDGE_CURVE ( 'NONE', #4873, #2508, #10085, .T. ) ;
#4697=CARTESIAN_POINT ( 'NONE',  ( -24.98076211353213694, 57.86529025992057029, -6.732050807568382922 ) ) ;
#4711=CARTESIAN_POINT ( 'NONE',  ( -27.98076211353308551, 51.30833333333320212, -3.845299461620869330 ) ) ;
#4712=CARTESIAN_POINT ( 'NONE',  ( -27.60187600103308014, 51.58541666571061768, -5.935950539335252074 ) ) ;
#4725=DIRECTION ( 'NONE',  ( 0.000000000000000000, 0.000000000000000000, 1.000000000000000000 ) ) ;
#4726=CIRCLE ( 'NONE', #9501, 3.500000000000591971 ) ;
#4727=CARTESIAN_POINT ( 'NONE',  ( -24.35964822603314772, 51.17708333237728624, -5.935950539335252074 ) ) ;
#4730=CARTESIAN_POINT ( 'NONE',  ( -25.98076211353311393, 54.96874999904394343, -6.871901078670400231 ) ) ;
#4731=EDGE_CURVE ( 'NONE', #4732, #6644, #9, .T. ) ;
#4732=VERTEX_POINT ( 'NONE', #4256 ) ;
#4733=DIRECTION ( 'NONE',  ( 0.000000000000000000, 1.000000000000000000, 0.000000000000000000 ) ) ;
#4738=VERTEX_POINT ( 'NONE', #10024 ) ;
#4746=CARTESIAN_POINT ( 'NONE',  ( -23.98076211353314235, 52.27083333142136468, -6.154700538379337615 ) ) ;
#4747=CARTESIAN_POINT ( 'NONE',  ( -26.51666049839535688, 53.20626073911682141, -7.000000000000071942 ) ) ;
#4753=( BOUNDED_CURVE ( )  B_SPLINE_CURVE ( 2, ( #399, #7974, #2024, #3799, #8076, #9022, #1411 ),
 .UNSPECIFIED., .F., .F. ) 
 B_SPLINE_CURVE_WITH_KNOTS ( ( 3, 2, 2, 3 ),
 ( 0.9166666666666666297, 0.9259259259259259300, 0.9444444444444444198, 0.9524107084371162824 ),
 .UNSPECIFIED. ) 
 CURVE ( )  GEOMETRIC_REPRESENTATION_ITEM ( )  RATIONAL_B_SPLINE_CURVE ( ( 0.9330127018922194093, 0.9330127018922189652, 1.000000000000000000, 0.8660254037844387076, 1.000000000000000000, 0.9423670419047019964, 0.9343189745669037150 ) ) 
 REPRESENTATION_ITEM ( '' )  );
#4761=DIRECTION ( 'NONE',  ( 0.000000000000000000, 0.000000000000000000, 1.000000000000000000 ) ) ;
#4769=CARTESIAN_POINT ( 'NONE',  ( -27.60187600103308014, 50.88541666571062194, -5.935950539335252074 ) ) ;
#4774=CARTESIAN_POINT ( 'NONE',  ( -25.44486372867087454, 54.16876073720499818, -3.000000000000134559 ) ) ;
#4775=FACE_OUTER_BOUND ( 'NONE', #1918, .T. ) ;
#4789=ORIENTED_EDGE ( 'NONE', *, *, #9452, .T. ) ;
#4792=ADVANCED_FACE ( 'NONE', ( #7971 ), #5254, .T. ) ;
#4796=CARTESIAN_POINT ( 'NONE',  ( -25.98076211353311393, 52.73749999808804034, -2.690598923241634743 ) ) ;
#4818=CARTESIAN_POINT ( 'NONE',  ( -25.17020516978313083, 51.70208333237728482, -3.596074190997380349 ) ) ;
#4822=AXIS2_PLACEMENT_3D ( 'NONE', #2704, #1022, #3589 ) ;
#4829=CARTESIAN_POINT ( 'NONE',  ( -24.35964822603314417, 53.21874999904395764, -5.000000000000103029 ) ) ;
#4831=CARTESIAN_POINT ( 'NONE',  ( -25.17020516978313083, 55.43541666571061910, -6.403925809002825709 ) ) ;
#4833=CARTESIAN_POINT ( 'NONE',  ( -27.60187600103308725, 55.86681146796335895, -4.629981812462977686 ) ) ;
#4844=CARTESIAN_POINT ( 'NONE',  ( -23.98076211353314235, 50.17083333142137036, -6.154700538379337615 ) ) ;
#4850=EDGE_CURVE ( 'NONE', #101, #10992, #3689, .T. ) ;
#4852=ADVANCED_FACE ( 'NONE', ( #9688 ), #7813, .T. ) ;
#4853=CARTESIAN_POINT ( 'NONE',  ( -25.98076211353311393, 49.49999999999986500, -3.000000000000131894 ) ) ;
#4861=VERTEX_POINT ( 'NONE', #1183 ) ;
#4865=CARTESIAN_POINT ( 'NONE',  ( -23.98076211353314235, 50.11249999808803324, -5.000000000000103029 ) ) ;
#4869=CARTESIAN_POINT ( 'NONE',  ( -26.79131905728310059, 55.02708333237728056, -6.403925809002825709 ) ) ;
#4873=VERTEX_POINT ( 'NONE', #6076 ) ;
#4879=CARTESIAN_POINT ( 'NONE',  ( -25.98076211353310683, 51.99374999904394912, -6.871901078670399343 ) ) ;
#4882=CARTESIAN_POINT ( 'NONE',  ( -25.98076211353311393, 50.37499999999986500, -7.309401076758571314 ) ) ;
#4886=ADVANCED_FACE ( 'NONE', ( #2701 ), #9466, .T. ) ;
#4903=CARTESIAN_POINT ( 'NONE',  ( -24.98076211353312814, 52.32916666475470180, -6.732050807568954909 ) ) ;
#4922=ORIENTED_EDGE ( 'NONE', *, *, #1796, .T. ) ;
#4929=CARTESIAN_POINT ( 'NONE',  ( -25.98076211353311749, 56.99999999999884182, -7.000000000000094147 ) ) ;
#4931=CARTESIAN_POINT ( 'NONE',  ( -27.60187600103308370, 55.84374999904394343, -5.000000000000103029 ) ) ;
#4939=CARTESIAN_POINT ( 'NONE',  ( -27.98076211353308551, 50.54999999999986926, -5.000000000000103029 ) ) ;
#4940=CARTESIAN_POINT ( 'NONE',  ( -24.35964822603314772, 51.35208333237727629, -5.935950539335252074 ) ) ;
#4941=CARTESIAN_POINT ( 'NONE',  ( -26.79131905728310059, 52.28541666571062052, -3.596074190997381237 ) ) ;
#4943=B_SPLINE_CURVE_WITH_KNOTS ( 'NONE', 3,
 ( #10370, #1260, #8819, #3811, #5431, #7934, #357, #3706, #251, #199 ),
 .UNSPECIFIED., .F., .F.,
 ( 4, 2, 2, 2, 4 ),
 ( 0.001590949097579384165, 0.001988361050532979398, 0.002385773003486574631, 0.002783184956440169864, 0.003180596909393765097 ),
 .UNSPECIFIED. ) ;
#4946=CARTESIAN_POINT ( 'NONE',  ( -26.98076211353309972, 52.76666666666653072, -3.267949192431252037 ) ) ;
#4952=ORIENTED_EDGE ( 'NONE', *, *, #9594, .T. ) ;
#4962=CARTESIAN_POINT ( 'NONE',  ( -26.98076211353309972, 53.37916666475469896, -3.267949192431252037 ) ) ;
#4963=CARTESIAN_POINT ( 'NONE',  ( -27.98076211353308551, 53.34999999999985931, -5.000000000000103029 ) ) ;
#4964=CARTESIAN_POINT ( 'NONE',  ( -26.51666049839535688, 51.01876073720499960, -7.000000000000074607 ) ) ;
#4979=CARTESIAN_POINT ( 'NONE',  ( -27.98076211353308551, 54.66249999808803040, -5.000000000000103029 ) ) ;
#4983=CARTESIAN_POINT ( 'NONE',  ( -26.79131905728310059, 55.72708333237728340, -6.403925809002825709 ) ) ;
#4990=EDGE_CURVE ( 'NONE', #1598, #4566, #8965, .T. ) ;
#4991=CARTESIAN_POINT ( 'NONE',  ( -26.79131905728310059, 50.12708333237728198, -6.403925809002825709 ) ) ;
#4992=CARTESIAN_POINT ( 'NONE',  ( -26.79131905728310059, 54.38541666571061484, -3.596074190997381237 ) ) ;
#4995=CARTESIAN_POINT ( 'NONE',  ( -27.98076211353308551, 52.59166666666653356, -6.154700538379338504 ) ) ;
#5004=VERTEX_POINT ( 'NONE', #30 ) ;
#5012=CARTESIAN_POINT ( 'NONE',  ( -23.98076211353314235, 54.95416666475470180, -3.845299461620867554 ) ) ;
#5020=ORIENTED_EDGE ( 'NONE', *, *, #6532, .F. ) ;
#5028=CARTESIAN_POINT ( 'NONE',  ( -25.98076211353311393, 51.68749999808803608, -7.000000000000073719 ) ) ;
#5035=CARTESIAN_POINT ( 'NONE',  ( -23.98076211353314235, 55.71249999808803466, -5.000000000000103029 ) ) ;
#5037=CARTESIAN_POINT ( 'NONE',  ( -26.79131905728310059, 50.88541666571061484, -3.596074190997381237 ) ) ;
#5041=( BOUNDED_CURVE ( )  B_SPLINE_CURVE ( 2, ( #7363, #3923, #7308, #10544, #7205, #4660, #9871 ),
 .UNSPECIFIED., .F., .F. ) 
 B_SPLINE_CURVE_WITH_KNOTS ( ( 3, 2, 2, 3 ),
 ( 0.9166666666666667407, 0.9259259259259259300, 0.9444444444444444198, 0.9524110019352027834 ),
 .UNSPECIFIED. ) 
 CURVE ( )  GEOMETRIC_REPRESENTATION_ITEM ( )  RATIONAL_B_SPLINE_CURVE ( ( 0.9330127018922194093, 0.9330127018922197424, 1.000000000000000000, 0.8660254037844387076, 1.000000000000000000, 0.9423649185551699059, 0.9343183816103359796 ) ) 
 REPRESENTATION_ITEM ( '' )  );
#5045=CARTESIAN_POINT ( 'NONE',  ( -26.79131905728310059, 55.72708333237728340, -6.403925809002825709 ) ) ;
#5047=CARTESIAN_POINT ( 'NONE',  ( -27.44132332507749794, 55.71836679508493262, -4.296600267573891685 ) ) ;
#5049=CARTESIAN_POINT ( 'NONE',  ( -23.98076211353314235, 51.54166666666652219, -3.845299461620867554 ) ) ;
#5065=CARTESIAN_POINT ( 'NONE',  ( -27.60187600103308014, 50.30208333237727913, -4.064049460664955760 ) ) ;
#5068=CARTESIAN_POINT ( 'NONE',  ( -24.35964822603314772, 49.95208333237727771, -5.935950539335252074 ) ) ;
#5072=CARTESIAN_POINT ( 'NONE',  ( -27.98076211353308551, 50.40416666475469754, -6.154700538379338504 ) ) ;
#5079=VECTOR ( 'NONE', #5362, 1000.000000000000000 ) ;
#5080=CARTESIAN_POINT ( 'NONE',  ( -25.00815916299270825, 58.26638652017265940, -6.748499677373088979 ) ) ;
#5082=CARTESIAN_POINT ( 'NONE',  ( -25.17020516978313083, 51.70208333237728482, -3.596074190997380349 ) ) ;
#5084=CARTESIAN_POINT ( 'NONE',  ( -25.98076211353311393, 51.33749999808802755, -3.000000000000132783 ) ) ;
#5089=CYLINDRICAL_SURFACE ( 'NONE', #6490, 1.999999999999971356 ) ;
#5095=CARTESIAN_POINT ( 'NONE',  ( -27.60187600103308014, 53.51041666571062194, -5.935950539335252074 ) ) ;
#5104=CARTESIAN_POINT ( 'NONE',  ( -27.60187600103308725, 52.40208333237728056, -4.064049460664955760 ) ) ;
#5106=( BOUNDED_CURVE ( )  B_SPLINE_CURVE ( 2, ( #7185, #9852, #10584, #6401, #9796, #2185, #5581, #1357, #10011 ),
 .UNSPECIFIED., .F., .F. ) 
 B_SPLINE_CURVE_WITH_KNOTS ( ( 3, 2, 2, 2, 3 ),
 ( 0.02777777777777775542, 0.03703703703703703498, 0.05555555555555555247, 0.07407407407407406996, 0.08333333333333331483 ),
 .UNSPECIFIED. ) 
 CURVE ( )  GEOMETRIC_REPRESENTATION_ITEM ( )  RATIONAL_B_SPLINE_CURVE ( ( 0.9330127018922194093, 0.9330127018922191873, 1.000000000000000000, 0.8660254037844387076, 1.000000000000000000, 0.8660254037844387076, 1.000000000000000000, 0.9330127018922194093, 0.9330127018922192983 ) ) 
 REPRESENTATION_ITEM ( '' )  );
#5110=CARTESIAN_POINT ( 'NONE',  ( -27.98076211353308551, 54.10833333333319217, -3.845299461620869330 ) ) ;
#5117=ORIENTED_EDGE ( 'NONE', *, *, #3582, .T. ) ;
#5122=CARTESIAN_POINT ( 'NONE',  ( -26.98076211353309972, 51.74583333142136610, -6.732050807568954909 ) ) ;
#5123=CARTESIAN_POINT ( 'NONE',  ( -23.98076211353314235, 50.11249999808803324, -5.000000000000103029 ) ) ;
#5126=CARTESIAN_POINT ( 'NONE',  ( -24.98076211353313170, 54.89583333142136468, -3.267949192431250705 ) ) ;
#5131=ORIENTED_EDGE ( 'NONE', *, *, #2967, .T. ) ;
#5137=EDGE_CURVE ( 'NONE', #6171, #10078, #6114, .T. ) ;
#5140=CARTESIAN_POINT ( 'NONE',  ( -27.60187600103308014, 50.12708333237727487, -4.064049460664955760 ) ) ;
#5149=CARTESIAN_POINT ( 'NONE',  ( -26.51666049839534978, 54.80623925897107540, -3.000000000000133227 ) ) ;
#5153=CARTESIAN_POINT ( 'NONE',  ( -26.79131905728310059, 52.28541666571062052, -3.596074190997381237 ) ) ;
#5160=CARTESIAN_POINT ( 'NONE',  ( -24.35964822603314772, 54.15208333237727345, -5.935950539335252074 ) ) ;
#5161=EDGE_CURVE ( 'NONE', #5523, #9017, #5347, .T. ) ;
#5162=CARTESIAN_POINT ( 'NONE',  ( -24.98076211353312814, 51.01666666666653072, -6.732050807568954909 ) ) ;
#5164=CARTESIAN_POINT ( 'NONE',  ( -27.98076211353308551, 51.89166666666653782, -6.154700538379338504 ) ) ;
#5170=ORIENTED_EDGE ( 'NONE', *, *, #1042, .T. ) ;
#5171=DIRECTION ( 'NONE',  ( 0.000000000000000000, -1.000000000000000000, 0.000000000000000000 ) ) ;
#5173=CARTESIAN_POINT ( 'NONE',  ( -26.98076211353309972, 51.97916666475470038, -3.267949192431252037 ) ) ;
#5177=CARTESIAN_POINT ( 'NONE',  ( -23.98076211353314235, 54.37083333142137320, -6.154700538379337615 ) ) ;
#5179=CARTESIAN_POINT ( 'NONE',  ( -23.98076211353314235, 53.69999999999986784, -5.000000000000103029 ) ) ;
#5181=CARTESIAN_POINT ( 'NONE',  ( -26.51666049839534622, 50.60623925897106545, -3.000000000000131006 ) ) ;
#5189=CARTESIAN_POINT ( 'NONE',  ( -26.79131905728310059, 52.98541666571061626, -3.596074190997381237 ) ) ;
#5203=VECTOR ( 'NONE', #178, 1000.000000000000000 ) ;
#5204=CARTESIAN_POINT ( 'NONE',  ( -25.44486372867087454, 55.56876073720499676, -3.000000000000134559 ) ) ;
#5205=CARTESIAN_POINT ( 'NONE',  ( -25.98076211353311393, 59.00000000000083134, -7.000000000000074607 ) ) ;
#5206=CARTESIAN_POINT ( 'NONE',  ( -27.60187600103308370, 53.56874999904395196, -5.000000000000103029 ) ) ;
#5208=CARTESIAN_POINT ( 'NONE',  ( -25.47250412700868338, 57.12887987407799528, -3.061742751175442923 ) ) ;
#5213=CARTESIAN_POINT ( 'NONE',  ( -26.51666049839534978, 54.19373926088289295, -3.000000000000133227 ) ) ;
#5216=CARTESIAN_POINT ( 'NONE',  ( -26.79131905728310059, 52.22708333237727629, -6.403925809002825709 ) ) ;
#5217=CARTESIAN_POINT ( 'NONE',  ( -24.35964822603314417, 55.31874999904395196, -5.000000000000103029 ) ) ;
#5231=CARTESIAN_POINT ( 'NONE',  ( -25.17020516978313083, 50.47708333237727629, -3.596074190997380349 ) ) ;
#5243=CARTESIAN_POINT ( 'NONE',  ( -24.35964822603314772, 51.06041666571061199, -4.064049460664953983 ) ) ;
#5252=DIRECTION ( 'NONE',  ( 0.000000000000000000, 1.000000000000000000, 0.000000000000000000 ) ) ;
#5254=CYLINDRICAL_SURFACE ( 'NONE', #3286, 1.999999999999971356 ) ;
#5257=CARTESIAN_POINT ( 'NONE',  ( -25.98076211353311393, 52.82499999999986784, -3.000000000000132339 ) ) ;
#5259=CARTESIAN_POINT ( 'NONE',  ( -27.60187600103308014, 55.02708333237728056, -4.064049460664955760 ) ) ;
#5263=CARTESIAN_POINT ( 'NONE',  ( -26.98076211353309972, 54.07916666475470180, -3.267949192431252037 ) ) ;
#5267=CARTESIAN_POINT ( 'NONE',  ( -25.98076211353310683, 53.91874999904394627, -3.128098921329806714 ) ) ;
#5276=ORIENTED_EDGE ( 'NONE', *, *, #1740, .F. ) ;
#5283=SHAPE_REPRESENTATION ( 'Cable Pinch Bolt Clamp', ( #308 ), #6179 ) ;
#5286=CARTESIAN_POINT ( 'NONE',  ( -25.98076211353311393, 53.21874999904395054, -3.128098921329806714 ) ) ;
#5299=DIRECTION ( 'NONE',  ( 0.000000000000000000, 1.000000000000000000, 0.000000000000000000 ) ) ;
#5302=CARTESIAN_POINT ( 'NONE',  ( -25.17020516978313083, 51.23541666571061626, -6.403925809002825709 ) ) ;
#5312=CARTESIAN_POINT ( 'NONE',  ( -26.95345029339875609, 58.26591186299814495, -3.251555783389634247 ) ) ;
#5314=CARTESIAN_POINT ( 'NONE',  ( -27.60187600103308014, 52.81041666571061199, -5.935950539335252074 ) ) ;
#5315=CARTESIAN_POINT ( 'NONE',  ( -23.98076211353314235, 49.55833333333319501, -6.154700538379337615 ) ) ;
#5322=UNCERTAINTY_MEASURE_WITH_UNIT (LENGTH_MEASURE( 1.000000000000000082E-05 ), #3894, 'distance_accuracy_value', 'NONE');
#5324=CARTESIAN_POINT ( 'NONE',  ( -23.98076211353314235, 52.99999999999986500, -5.000000000000103029 ) ) ;
#5331=LINE ( 'NONE', #5441, #3274 ) ;
#5338=CARTESIAN_POINT ( 'NONE',  ( -24.35964822603314417, 52.69374999904394485, -5.000000000000103029 ) ) ;
#5347=( BOUNDED_CURVE ( )  B_SPLINE_CURVE ( 2, ( #6037, #8591, #9252, #8419, #801, #6754, #9585, #8816, #1935 ),
 .UNSPECIFIED., .F., .F. ) 
 B_SPLINE_CURVE_WITH_KNOTS ( ( 3, 2, 2, 2, 3 ),
 ( 0.4722222222222222099, 0.4814814814814814548, 0.5000000000000000000, 0.5185185185185184897, 0.5277777777777777901 ),
 .UNSPECIFIED. ) 
 CURVE ( )  GEOMETRIC_REPRESENTATION_ITEM ( )  RATIONAL_B_SPLINE_CURVE ( ( 0.9330127018922194093, 0.9330127018922194093, 1.000000000000000000, 0.8660254037844387076, 1.000000000000000000, 0.8660254037844387076, 1.000000000000000000, 0.9330127018922194093, 0.9330127018922194093 ) ) 
 REPRESENTATION_ITEM ( '' )  );
#5351=CARTESIAN_POINT ( 'NONE',  ( -25.17020516978313083, 53.80208333237728624, -3.596074190997380349 ) ) ;
#5355=CARTESIAN_POINT ( 'NONE',  ( -25.98076211353311393, 49.49999999999986500, -5.000000000000103029 ) ) ;
#5362=DIRECTION ( 'NONE',  ( 0.000000000000000000, 1.000000000000000000, 0.000000000000000000 ) ) ;
#5368=ORIENTED_EDGE ( 'NONE', *, *, #9673, .T. ) ;
#5375=CARTESIAN_POINT ( 'NONE',  ( -24.35964822603314772, 53.45208333237727771, -5.935950539335252074 ) ) ;
#5377=CARTESIAN_POINT ( 'NONE',  ( -26.98076211353309972, 54.63333333333319786, -6.732050807568954909 ) ) ;
#5382=DIRECTION ( 'NONE',  ( 0.000000000000000000, 0.000000000000000000, 1.000000000000000000 ) ) ;
#5391=CARTESIAN_POINT ( 'NONE',  ( -26.79131905728310059, 52.46041666571061768, -3.596074190997381237 ) ) ;
#5403=ADVANCED_FACE ( 'NONE', ( #288 ), #4208, .T. ) ;
#5405=CARTESIAN_POINT ( 'NONE',  ( -27.60187600103308014, 53.51041666571062194, -5.935950539335252074 ) ) ;
#5408=CARTESIAN_POINT ( 'NONE',  ( -24.98076211353313170, 52.79583333142137036, -3.267949192431250705 ) ) ;
#5410=( BOUNDED_CURVE ( )  B_SPLINE_CURVE ( 2, ( #1326, #3776, #4668, #325, #3828, #9826, #7214, #4618, #2163, #3053, #3721, #10505, #2895, #3882, #6264, #10607, #9658, #2054, #2212, #7266, #8003, #5610, #3005, #6383, #8935, #4727, #8104, #482, #8993, #1383, #3151, #643, #3200, #6637, #533, #1650, #5872, #1539, #8157, #4879, #6580, #5817, #7373, #10816, #4941, #8259, #4039, #9982, #7426, #10101, #9255, #6702, #2367, #1482, #5760, #3932, #8204, #6535, #2487, #2428, #4829, #10759, #9143, #9932, #8313, #9879, #7316, #2317, #695, #4093, #7481, #10869, #5708, #3258, #9088, #10042, #9202, #1595, #584, #10705, #4992, #2270, #8366, #745, #4145, #7537, #10926, #3100, #3318, #6479, #5662, #9041, #1432, #3979, #9538, #32, #5217, #868, #8594, #7656, #10987, #9481, #1879, #8484, #5047 ),
 .UNSPECIFIED., .F., .F. ) 
 B_SPLINE_CURVE_WITH_KNOTS ( ( 3, 2, 2, 2, 2, 2, 2, 2, 2, 2, 2, 2, 2, 2, 2, 2, 2, 2, 2, 2, 2, 2, 2, 2, 2, 2, 2, 2, 2, 2, 2, 2, 2, 2, 2, 2, 2, 2, 2, 2, 2, 2, 2, 2, 2, 2, 2, 2, 2, 2, 2, 2, 3 ),
 ( 0.000000000000000000, 0.01851851851851851749, 0.03703703703703703498, 0.05555555555555555247, 0.07407407407407406996, 0.09259259259259258745, 0.1111111111111111049, 0.1296296296296296224, 0.1481481481481481399, 0.1666666666666666574, 0.1851851851851851749, 0.2037037037037036924, 0.2222222222222222099, 0.2407407407407407274, 0.2592592592592592449, 0.2777777777777777901, 0.2962962962962962798, 0.3148148148148148806, 0.3333333333333333148, 0.3518518518518518601, 0.3703703703703703498, 0.3888888888888888951, 0.4074074074074073848, 0.4259259259259259300, 0.4444444444444444198, 0.4629629629629629650, 0.4814814814814814548, 0.5000000000000000000, 0.5185185185185184897, 0.5370370370370370905, 0.5555555555555555802, 0.5740740740740740700, 0.5925925925925925597, 0.6111111111111111605, 0.6296296296296297612, 0.6481481481481481399, 0.6666666666666666297, 0.6851851851851852304, 0.7037037037037037202, 0.7222222222222222099, 0.7407407407407406996, 0.7592592592592594114, 0.7777777777777777901, 0.7962962962962962798, 0.8148148148148147696, 0.8333333333333333703, 0.8518518518518518601, 0.8703703703703703498, 0.8888888888888888395, 0.9074074074074074403, 0.9259259259259259300, 0.9444444444444444198, 0.9524110019551521589 ),
 .UNSPECIFIED. ) 
 CURVE ( )  GEOMETRIC_REPRESENTATION_ITEM ( )  RATIONAL_B_SPLINE_CURVE ( ( 1.000000000000000000, 0.8660254037844387076, 1.000000000000000000, 0.8660254037844387076, 1.000000000000000000, 0.8660254037844387076, 1.000000000000000000, 0.8660254037844387076, 1.000000000000000000, 0.8660254037844387076, 1.000000000000000000, 0.8660254037844387076, 1.000000000000000000, 0.8660254037844387076, 1.000000000000000000, 0.8660254037844387076, 1.000000000000000000, 0.8660254037844387076, 1.000000000000000000, 0.8660254037844387076, 1.000000000000000000, 0.8660254037844387076, 1.000000000000000000, 0.8660254037844387076, 1.000000000000000000, 0.8660254037844387076, 1.000000000000000000, 0.8660254037844387076, 1.000000000000000000, 0.8660254037844387076, 1.000000000000000000, 0.8660254037844387076, 1.000000000000000000, 0.8660254037844387076, 1.000000000000000000, 0.8660254037844387076, 1.000000000000000000, 0.8660254037844387076, 1.000000000000000000, 0.8660254037844387076, 1.000000000000000000, 0.8660254037844387076, 1.000000000000000000, 0.8660254037844387076, 1.000000000000000000, 0.8660254037844387076, 1.000000000000000000, 0.8660254037844387076, 1.000000000000000000, 0.8660254037844387076, 1.000000000000000000, 0.8660254037844387076, 1.000000000000000000, 0.8660254037844387076, 1.000000000000000000, 0.8660254037844387076, 1.000000000000000000, 0.8660254037844387076, 1.000000000000000000, 0.8660254037844387076, 1.000000000000000000, 0.8660254037844387076, 1.000000000000000000, 0.8660254037844387076, 1.000000000000000000, 0.8660254037844387076, 1.000000000000000000, 0.8660254037844387076, 1.000000000000000000, 0.8660254037844387076, 1.000000000000000000, 0.8660254037844387076, 1.000000000000000000, 0.8660254037844387076, 1.000000000000000000, 0.8660254037844387076, 1.000000000000000000, 0.8660254037844387076, 1.000000000000000000, 0.8660254037844387076, 1.000000000000000000, 0.8660254037844387076, 1.000000000000000000, 0.8660254037844387076, 1.000000000000000000, 0.8660254037844387076, 1.000000000000000000, 0.8660254037844387076, 1.000000000000000000, 0.8660254037844387076, 1.000000000000000000, 0.8660254037844387076, 1.000000000000000000, 0.8660254037844387076, 1.000000000000000000, 0.8660254037844387076, 1.000000000000000000, 0.8660254037844387076, 1.000000000000000000, 0.8660254037844387076, 1.000000000000000000, 0.8660254037844387076, 1.000000000000000000, 0.9423649184108428001, 0.9343183815700366601 ) ) 
 REPRESENTATION_ITEM ( '' )  );
#5418=CARTESIAN_POINT ( 'NONE',  ( -26.51666049839535333, 52.70623925897106687, -3.000000000000132339 ) ) ;
#5421=( NAMED_UNIT ( * ) SI_UNIT ( $, .STERADIAN. ) SOLID_ANGLE_UNIT ( ) );
#5431=CARTESIAN_POINT ( 'NONE',  ( -26.59870219654672141, 57.20337143919491041, -6.904607032842216441 ) ) ;
#5435=CARTESIAN_POINT ( 'NONE',  ( -24.35964822603314772, 51.23541666571061626, -4.064049460664953983 ) ) ;
#5438=ORIENTED_EDGE ( 'NONE', *, *, #6361, .T. ) ;
#5439=ORIENTED_EDGE ( 'NONE', *, *, #6409, .F. ) ;
#5441=CARTESIAN_POINT ( 'NONE',  ( -25.98076211353311393, 49.49999999999986500, -7.000000000000074607 ) ) ;
#5449=CARTESIAN_POINT ( 'NONE',  ( -24.35964822603314772, 54.03541666571061342, -4.064049460664953983 ) ) ;
#5455=ORIENTED_EDGE ( 'NONE', *, *, #1537, .F. ) ;
#5460=CARTESIAN_POINT ( 'NONE',  ( -24.98076211353312814, 49.61666666666653214, -6.732050807568954909 ) ) ;
#5475=CARTESIAN_POINT ( 'NONE',  ( -26.11341725377009482, 59.00000000000061107, -3.000000000000243805 ) ) ;
#5476=( GEOMETRIC_REPRESENTATION_CONTEXT ( 3 ) GLOBAL_UNCERTAINTY_ASSIGNED_CONTEXT ( ( #8083 ) ) GLOBAL_UNIT_ASSIGNED_CONTEXT ( ( #4537, #6976, #5421 ) ) REPRESENTATION_CONTEXT ( 'NONE', 'WORKASPACE' ) );
#5491=CARTESIAN_POINT ( 'NONE',  ( -25.98076211353311393, 54.83749999808802755, -3.000000000000132339 ) ) ;
#5495=CARTESIAN_POINT ( 'NONE',  ( -27.60187600103308014, 51.70208333237727771, -4.064049460664955760 ) ) ;
#5499=DIRECTION ( 'NONE',  ( 0.000000000000000000, 1.000000000000000000, 0.000000000000000000 ) ) ;
#5507=CARTESIAN_POINT ( 'NONE',  ( -27.60187600103308370, 51.64374999904394770, -5.000000000000103029 ) ) ;
#5523=VERTEX_POINT ( 'NONE', #3886 ) ;
#5536=EDGE_CURVE ( 'NONE', #433, #3324, #9525, .T. ) ;
#5537=AXIS2_PLACEMENT_3D ( 'NONE', #9067, #10794, #1514 ) ;
#5543=CARTESIAN_POINT ( 'NONE',  ( -25.98076211353311393, 51.42499999999986926, -3.000000000000132339 ) ) ;
#5544=CARTESIAN_POINT ( 'NONE',  ( -25.17020516978313083, 51.17708333237727913, -3.596074190997380349 ) ) ;
#5549=DIRECTION ( 'NONE',  ( -0.000000000000000000, -0.000000000000000000, 1.000000000000000000 ) ) ;
#5553=CARTESIAN_POINT ( 'NONE',  ( -25.98076211353311393, 49.49999999999986500, -5.000000000000103029 ) ) ;
#5554=CARTESIAN_POINT ( 'NONE',  ( -25.98076211353311038, 61.49999999999985789, -8.500000000000694556 ) ) ;
#5561=FACE_OUTER_BOUND ( 'NONE', #507, .T. ) ;
#5572=CARTESIAN_POINT ( 'NONE',  ( -23.98076211353314235, 52.85416666475470748, -3.845299461620867554 ) ) ;
#5575=VERTEX_POINT ( 'NONE', #2824 ) ;
#5576=ORIENTED_EDGE ( 'NONE', *, *, #9957, .T. ) ;
#5581=CARTESIAN_POINT ( 'NONE',  ( -26.98076211353309972, 49.96666666666652645, -3.267949192431252037 ) ) ;
#5589=AXIS2_PLACEMENT_3D ( 'NONE', #8203, #7536, #2269 ) ;
#5595=CARTESIAN_POINT ( 'NONE',  ( -27.60187600103308014, 53.80208333237727203, -4.064049460664955760 ) ) ;
#5599=VERTEX_POINT ( 'NONE', #7139 ) ;
#5610=CARTESIAN_POINT ( 'NONE',  ( -25.98076211353310683, 50.94374999904394485, -3.128098921329806714 ) ) ;
#5614=CARTESIAN_POINT ( 'NONE',  ( -26.98076211353309972, 53.84583333142136752, -6.732050807568954909 ) ) ;
#5617=ORIENTED_EDGE ( 'NONE', *, *, #3686, .T. ) ;
#5626=CARTESIAN_POINT ( 'NONE',  ( -24.98076211353312814, 50.92916666475470322, -6.732050807568954909 ) ) ;
#5628=DIRECTION ( 'NONE',  ( 0.000000000000000000, -0.000000000000000000, 1.000000000000000000 ) ) ;
#5652=CARTESIAN_POINT ( 'NONE',  ( -27.60187600103308014, 51.52708333237728766, -4.064049460664955760 ) ) ;
#5657=AXIS2_PLACEMENT_3D ( 'NONE', #9135, #10032, #6417 ) ;
#5659=CARTESIAN_POINT ( 'NONE',  ( -25.98076211353311038, 57.99999999999985789, -9.000000000000701661 ) ) ;
#5661=CARTESIAN_POINT ( 'NONE',  ( -24.35964822603314417, 49.89374999904394770, -5.000000000000103029 ) ) ;
#5662=CARTESIAN_POINT ( 'NONE',  ( -27.60187600103308370, 54.96874999904395054, -5.000000000000103029 ) ) ;
#5664=CARTESIAN_POINT ( 'NONE',  ( -24.35964822603314772, 55.26041666571062194, -4.064049460664953983 ) ) ;
#5670=ORIENTED_EDGE ( 'NONE', *, *, #2748, .T. ) ;
#5678=CARTESIAN_POINT ( 'NONE',  ( -23.98076211353314235, 53.67083333142136325, -6.154700538379337615 ) ) ;
#5699=EDGE_CURVE ( 'NONE', #5575, #5004, #6504, .T. ) ;
#5701=CARTESIAN_POINT ( 'NONE',  ( -24.35964822603314417, 50.41874999904395338, -5.000000000000103029 ) ) ;
#5703=CARTESIAN_POINT ( 'NONE',  ( -26.98076211353408382, 57.99999999999985789, -6.732050807568389139 ) ) ;
#5707=CARTESIAN_POINT ( 'NONE',  ( -25.98076211353310683, 50.06874999904394485, -6.871901078670399343 ) ) ;
#5708=CARTESIAN_POINT ( 'NONE',  ( -24.35964822603314417, 53.91874999904395338, -5.000000000000103029 ) ) ;
#5711=CARTESIAN_POINT ( 'NONE',  ( -23.98076211353314235, 50.25833333333319075, -6.154700538379337615 ) ) ;
#5712=ORIENTED_EDGE ( 'NONE', *, *, #10610, .F. ) ;
#5714=CARTESIAN_POINT ( 'NONE',  ( -25.98076211353311393, 55.31874999904394485, -3.128098921329806714 ) ) ;
#5716=EDGE_LOOP ( 'NONE', ( #9886, #5117, #9939, #5455 ) ) ;
#5718=ORIENTED_EDGE ( 'NONE', *, *, #2819, .T. ) ;
#5719=PLANE ( 'NONE',  #10017 ) ;
#5728=CARTESIAN_POINT ( 'NONE',  ( -24.98076211353313170, 52.09583333142136752, -3.267949192431250705 ) ) ;
#5748=DIRECTION ( 'NONE',  ( 0.000000000000000000, 1.000000000000000000, 0.000000000000000000 ) ) ;
#5749=CARTESIAN_POINT ( 'NONE',  ( -27.60187600103308014, 55.86681177618367400, -4.629976867109323990 ) ) ;
#5756=DIRECTION ( 'NONE',  ( 2.775557561562891351E-17, 1.000000000000000000, -8.326672684688671588E-17 ) ) ;
#5759=CARTESIAN_POINT ( 'NONE',  ( -26.79131905728310059, 51.06041666571061199, -3.596074190997381237 ) ) ;
#5760=CARTESIAN_POINT ( 'NONE',  ( -27.60187600103308370, 52.86874999904394912, -5.000000000000103029 ) ) ;
#5762=CARTESIAN_POINT ( 'NONE',  ( -27.98076211353308551, 50.49166666666652503, -6.154700538379338504 ) ) ;
#5764=VERTEX_POINT ( 'NONE', #1633 ) ;
#5769=ORIENTED_EDGE ( 'NONE', *, *, #2417, .T. ) ;
#5778=CARTESIAN_POINT ( 'NONE',  ( -24.98076211353312814, 53.02916666475469754, -6.732050807568954909 ) ) ;
#5785=EDGE_CURVE ( 'NONE', #9280, #101, #9818, .T. ) ;
#5804=FACE_OUTER_BOUND ( 'NONE', #2490, .T. ) ;
#5805=CARTESIAN_POINT ( 'NONE',  ( -27.60187600103308014, 50.01041666571062194, -5.935950539335252074 ) ) ;
#5814=CARTESIAN_POINT ( 'NONE',  ( -27.98076211353308551, 54.04999999999986215, -5.000000000000103029 ) ) ;
#5816=CARTESIAN_POINT ( 'NONE',  ( -27.60187600103308725, 51.70208333237728482, -4.064049460664955760 ) ) ;
#5817=CARTESIAN_POINT ( 'NONE',  ( -27.60187600103308725, 52.11041666571061626, -5.935950539335252074 ) ) ;
#5819=MECHANICAL_DESIGN_GEOMETRIC_PRESENTATION_REPRESENTATION('',(#3691),#4419);
#5822=CARTESIAN_POINT ( 'NONE',  ( -26.98076211353309972, 51.83333333333319359, -6.732050807568954909 ) ) ;
#5835=LINE ( 'NONE', #6772, #3332 ) ;
#5838=CARTESIAN_POINT ( 'NONE',  ( -27.98076211353308551, 56.06249999808802897, -5.000000000000103029 ) ) ;
#5841=CARTESIAN_POINT ( 'NONE',  ( -25.98076211353311393, 49.49999999999986500, -5.000000000000103029 ) ) ;
#5848=DIRECTION ( 'NONE',  ( -0.000000000000000000, -0.000000000000000000, 1.000000000000000000 ) ) ;
#5851=CARTESIAN_POINT ( 'NONE',  ( -23.98076211353314235, 51.51249999808803182, -5.000000000000103029 ) ) ;
#5854=VERTEX_POINT ( 'NONE', #6511 ) ;
#5855=ORIENTED_EDGE ( 'NONE', *, *, #754, .T. ) ;
#5862=DIRECTION ( 'NONE',  ( 2.775557561562891351E-17, 1.000000000000000000, -8.326672684688671588E-17 ) ) ;
#5863=CARTESIAN_POINT ( 'NONE',  ( -27.60187600103308014, 54.50208333237726777, -4.064049460664955760 ) ) ;
#5866=CARTESIAN_POINT ( 'NONE',  ( -25.98076211353310683, 54.13749999808803182, -3.000000000000132339 ) ) ;
#5869=CARTESIAN_POINT ( 'NONE',  ( -25.98076211353311038, 61.49999999999985789, -5.000000000000102141 ) ) ;
#5870=CARTESIAN_POINT ( 'NONE',  ( -27.60187600103308725, 53.68541666571061199, -5.935950539335252074 ) ) ;
#5872=CARTESIAN_POINT ( 'NONE',  ( -24.35964822603314417, 51.81874999904395196, -5.000000000000103029 ) ) ;
#5874=CARTESIAN_POINT ( 'NONE',  ( -24.98076211353312814, 51.71666666666652645, -6.732050807568954909 ) ) ;
#5877=ADVANCED_FACE ( 'NONE', ( #3961 ), #9916, .T. ) ;
#5887=LINE ( 'NONE', #10114, #1922 ) ;
#5890=CARTESIAN_POINT ( 'NONE',  ( -27.98076211353308551, 53.96249999808803466, -5.000000000000103029 ) ) ;
#5892=CARTESIAN_POINT ( 'NONE',  ( -25.44486372867087454, 53.55626073911682994, -3.000000000000134559 ) ) ;
#5894=CARTESIAN_POINT ( 'NONE',  ( -27.98076211353308551, 50.52083333142136468, -3.845299461620869330 ) ) ;
#5898=ORIENTED_EDGE ( 'NONE', *, *, #3844, .T. ) ;
#5901=CARTESIAN_POINT ( 'NONE',  ( -25.18166448601221319, 58.61490192845000990, -6.836013269862629471 ) ) ;
#5904=CARTESIAN_POINT ( 'NONE',  ( -25.17020516978313083, 51.93541666571061910, -6.403925809002825709 ) ) ;
#5915=CARTESIAN_POINT ( 'NONE',  ( -25.98076211353311393, 59.49999999999985789, -5.000000000000103029 ) ) ;
#5916=CARTESIAN_POINT ( 'NONE',  ( -24.35964822603314772, 54.67708333237728624, -5.935950539335252074 ) ) ;
#5918=CARTESIAN_POINT ( 'NONE',  ( -25.36311752100827732, 57.20314267782387674, -3.095295627716787568 ) ) ;
#5919=FACE_OUTER_BOUND ( 'NONE', #8069, .T. ) ;
#5922=CARTESIAN_POINT ( 'NONE',  ( -25.17020516978313083, 53.51041666571060773, -6.403925809002825709 ) ) ;
#5926=CARTESIAN_POINT ( 'NONE',  ( -26.98076211353309972, 53.93333333333319501, -6.732050807568954909 ) ) ;
#5946=CARTESIAN_POINT ( 'NONE',  ( -27.60187600103308370, 50.24374999904394912, -5.000000000000103029 ) ) ;
#5950=CARTESIAN_POINT ( 'NONE',  ( -25.98076211353311393, 50.28749999808804461, -7.000000000000073719 ) ) ;
#5959=AXIS2_PLACEMENT_3D ( 'NONE', #3814, #9762, #10909 ) ;
#5960=CARTESIAN_POINT ( 'NONE',  ( -24.35964822603314772, 51.76041666571060773, -4.064049460664953983 ) ) ;
#5974=CARTESIAN_POINT ( 'NONE',  ( -24.35964822603314417, 54.61874999904395622, -5.000000000000103029 ) ) ;
#5976=CARTESIAN_POINT ( 'NONE',  ( -25.98076211353311393, 49.49999999999986500, -5.000000000000103029 ) ) ;
#5979=CARTESIAN_POINT ( 'NONE',  ( -26.51666049839535333, 50.69373926088290006, -3.000000000000132783 ) ) ;
#5981=CARTESIAN_POINT ( 'NONE',  ( -27.60187600103308370, 55.14374999904394059, -5.000000000000103029 ) ) ;
#5986=CARTESIAN_POINT ( 'NONE',  ( -23.98076211353314235, 53.64166666666653072, -3.845299461620867554 ) ) ;
#6004=CARTESIAN_POINT ( 'NONE',  ( -24.35964822603314772, 50.65208333237728056, -5.935950539335252074 ) ) ;
#6008=ORIENTED_EDGE ( 'NONE', *, *, #9335, .T. ) ;
#6011=VERTEX_POINT ( 'NONE', #6913 ) ;
#6017=CARTESIAN_POINT ( 'NONE',  ( -25.98076211353311393, 50.24374999904395622, -3.128098921329806714 ) ) ;
#6030=CARTESIAN_POINT ( 'NONE',  ( -27.60187600103308370, 54.26874999904394770, -5.000000000000103029 ) ) ;
#6032=CARTESIAN_POINT ( 'NONE',  ( -25.98076211353311749, 56.99999999999886313, -3.000000000000122569 ) ) ;
#6035=CARTESIAN_POINT ( 'NONE',  ( -25.98076211353310683, 54.13749999808803182, -3.000000000000132339 ) ) ;
#6036=CARTESIAN_POINT ( 'NONE',  ( -25.98076211353311038, 61.49999999999985789, -5.000000000000102141 ) ) ;
#6037=CARTESIAN_POINT ( 'NONE',  ( -25.98076211353311393, 53.08749999808803466, -7.000000000000072831 ) ) ;
#6039=CARTESIAN_POINT ( 'NONE',  ( -24.35964822603314772, 53.45208333237727771, -5.935950539335252074 ) ) ;
#6041=FACE_OUTER_BOUND ( 'NONE', #261, .T. ) ;
#6046=EDGE_LOOP ( 'NONE', ( #10377, #10219, #2191, #9817, #3937, #5670 ) ) ;
#6051=( BOUNDED_CURVE ( )  B_SPLINE_CURVE ( 2, ( #3606, #10546, #8764, #1041, #9711, #7941, #1947, #10327, #367 ),
 .UNSPECIFIED., .F., .F. ) 
 B_SPLINE_CURVE_WITH_KNOTS ( ( 3, 2, 2, 2, 3 ),
 ( 0.8055555555555555802, 0.8148148148148147696, 0.8333333333333333703, 0.8518518518518518601, 0.8611111111111111605 ),
 .UNSPECIFIED. ) 
 CURVE ( )  GEOMETRIC_REPRESENTATION_ITEM ( )  RATIONAL_B_SPLINE_CURVE ( ( 0.9330127018922194093, 0.9330127018922197424, 1.000000000000000000, 0.8660254037844387076, 1.000000000000000000, 0.8660254037844387076, 1.000000000000000000, 0.9330127018922189652, 0.9330127018922194093 ) ) 
 REPRESENTATION_ITEM ( '' )  );
#6054=CARTESIAN_POINT ( 'NONE',  ( -23.98076211353314235, 55.01249999808803182, -5.000000000000103029 ) ) ;
#6066=CARTESIAN_POINT ( 'NONE',  ( -24.35964822603314417, 50.41874999904395338, -5.000000000000103029 ) ) ;
#6072=EDGE_CURVE ( 'NONE', #3184, #2547, #10788, .T. ) ;
#6076=CARTESIAN_POINT ( 'NONE',  ( -25.98076211353311393, 52.73749999808803324, -3.000000000000132783 ) ) ;
#6079=CARTESIAN_POINT ( 'NONE',  ( -24.98076211353313170, 55.59583333142136752, -3.267949192431250705 ) ) ;
#6081=CARTESIAN_POINT ( 'NONE',  ( -25.17020516978313083, 52.63541666571061484, -6.403925809002825709 ) ) ;
#6083=CARTESIAN_POINT ( 'NONE',  ( -25.00806794893706453, 57.73399265161810945, -3.251554382635098772 ) ) ;
#6089=CARTESIAN_POINT ( 'NONE',  ( -27.60187600103308370, 53.04374999904394627, -5.000000000000103029 ) ) ;
#6090=CARTESIAN_POINT ( 'NONE',  ( -25.98076211353311393, 49.49999999999986500, -7.000000000000074607 ) ) ;
#6093=VERTEX_POINT ( 'NONE', #9683 ) ;
#6098=ORIENTED_EDGE ( 'NONE', *, *, #10009, .F. ) ;
#6101=CARTESIAN_POINT ( 'NONE',  ( -24.98076211353312814, 54.51666666666653072, -6.732050807568954909 ) ) ;
#6105=CARTESIAN_POINT ( 'NONE',  ( -25.98076211353311393, 52.16874999904393917, -6.871901078670400231 ) ) ;
#6114=( BOUNDED_CURVE ( )  B_SPLINE_CURVE ( 2, ( #7709, #10924, #3256, #7534, #5814, #2603, #3374, #5213, #85 ),
 .UNSPECIFIED., .F., .F. ) 
 B_SPLINE_CURVE_WITH_KNOTS ( ( 3, 2, 2, 2, 3 ),
 ( 0.6944444444444445308, 0.7037037037037037202, 0.7222222222222222099, 0.7407407407407406996, 0.7500000000000000000 ),
 .UNSPECIFIED. ) 
 CURVE ( )  GEOMETRIC_REPRESENTATION_ITEM ( )  RATIONAL_B_SPLINE_CURVE ( ( 0.9330127018922194093, 0.9330127018922197424, 1.000000000000000000, 0.8660254037844387076, 1.000000000000000000, 0.8660254037844387076, 1.000000000000000000, 0.9330127018922194093, 0.9330127018922194093 ) ) 
 REPRESENTATION_ITEM ( '' )  );
#6118=CARTESIAN_POINT ( 'NONE',  ( -24.35964822603314772, 51.17708333237728624, -5.935950539335252074 ) ) ;
#6124=CARTESIAN_POINT ( 'NONE',  ( -25.98076211353311393, 52.38749999808802471, -7.000000000000072831 ) ) ;
#6125=CARTESIAN_POINT ( 'NONE',  ( -26.48707796582369056, 58.87212001354424018, -6.938716998541621273 ) ) ;
#6126=ORIENTED_EDGE ( 'NONE', *, *, #10009, .T. ) ;
#6128=CARTESIAN_POINT ( 'NONE',  ( -25.98076211353311393, 49.49999999999986500, -5.000000000000103029 ) ) ;
#6130=CARTESIAN_POINT ( 'NONE',  ( -25.98076211353311393, 49.49999999999986500, -5.000000000000103029 ) ) ;
#6131=CARTESIAN_POINT ( 'NONE',  ( -24.98076211353312814, 50.31666666666652787, -6.732050807568954909 ) ) ;
#6134=CARTESIAN_POINT ( 'NONE',  ( -24.35964822603314772, 52.57708333237728482, -5.935950539335252074 ) ) ;
#6155=EDGE_CURVE ( 'NONE', #4873, #5523, #2293, .T. ) ;
#6166=CARTESIAN_POINT ( 'NONE',  ( -24.35964822603314417, 54.09374999904395054, -5.000000000000103029 ) ) ;
#6171=VERTEX_POINT ( 'NONE', #9739 ) ;
#6179=( GEOMETRIC_REPRESENTATION_CONTEXT ( 3 ) GLOBAL_UNCERTAINTY_ASSIGNED_CONTEXT ( ( #6983 ) ) GLOBAL_UNIT_ASSIGNED_CONTEXT ( ( #3841, #1287, #9836 ) ) REPRESENTATION_CONTEXT ( 'NONE', 'WORKASPACE' ) );
#6181=CARTESIAN_POINT ( 'NONE',  ( -24.35964822603314772, 53.16041666571062763, -4.064049460664953983 ) ) ;
#6196=DIRECTION ( 'NONE',  ( 0.000000000000000000, -1.000000000000000000, 0.000000000000000000 ) ) ;
#6204=CARTESIAN_POINT ( 'NONE',  ( -25.98076211353311393, 53.21874999904395054, -3.128098921329806714 ) ) ;
#6206=DIRECTION ( 'NONE',  ( 0.000000000000000000, 0.000000000000000000, 1.000000000000000000 ) ) ;
#6209=CARTESIAN_POINT ( 'NONE',  ( -25.44486372867087454, 50.95623925897108109, -7.000000000000073719 ) ) ;
#6214=ADVANCED_FACE ( 'NONE', ( #232 ), #3628, .T. ) ;
#6219=CARTESIAN_POINT ( 'NONE',  ( -25.98076211353311393, 52.51874999904395480, -3.128098921329806714 ) ) ;
#6225=ORIENTED_EDGE ( 'NONE', *, *, #10443, .F. ) ;
#6229=CARTESIAN_POINT ( 'NONE',  ( -24.35964822603314417, 54.61874999904395622, -5.000000000000103029 ) ) ;
#6233=CARTESIAN_POINT ( 'NONE',  ( -24.98076211353312814, 50.22916666475470038, -6.732050807568954909 ) ) ;
#6237=CARTESIAN_POINT ( 'NONE',  ( -25.98076211353311393, 49.49999999999986500, -5.000000000000103029 ) ) ;
#6254=CARTESIAN_POINT ( 'NONE',  ( -27.60187600103308370, 51.64374999904394770, -5.000000000000103029 ) ) ;
#6257=ORIENTED_EDGE ( 'NONE', *, *, #9452, .F. ) ;
#6260=DIRECTION ( 'NONE',  ( -2.775557561562891351E-17, -1.000000000000000000, 8.326672684688671588E-17 ) ) ;
#6264=CARTESIAN_POINT ( 'NONE',  ( -25.17020516978313083, 50.53541666571062052, -6.403925809002825709 ) ) ;
#6269=CARTESIAN_POINT ( 'NONE',  ( -27.60187600103308370, 54.44374999904394485, -5.000000000000103029 ) ) ;
#6280=EDGE_CURVE ( 'NONE', #4274, #6817, #6462, .T. ) ;
#6281=CARTESIAN_POINT ( 'NONE',  ( -26.79131905728310059, 53.68541666571061910, -3.596074190997381237 ) ) ;
#6285=ORIENTED_EDGE ( 'NONE', *, *, #2110, .T. ) ;
#6287=ORIENTED_EDGE ( 'NONE', *, *, #8168, .T. ) ;
#6290=DIRECTION ( 'NONE',  ( 0.000000000000000000, 0.000000000000000000, 1.000000000000000000 ) ) ;
#6291=CARTESIAN_POINT ( 'NONE',  ( -25.98076211353311393, 53.43749999808803608, -3.000000000000132339 ) ) ;
#6312=CARTESIAN_POINT ( 'NONE',  ( -24.98076211353313170, 52.88333333333319786, -3.267949192431250705 ) ) ;
#6315=CARTESIAN_POINT ( 'NONE',  ( -24.35964822603314417, 51.99374999904394201, -5.000000000000103029 ) ) ;
#6320=DIRECTION ( 'NONE',  ( 0.000000000000000000, 1.000000000000000000, 0.000000000000000000 ) ) ;
#6322=ORIENTED_EDGE ( 'NONE', *, *, #9496, .T. ) ;
#6328=CARTESIAN_POINT ( 'NONE',  ( -25.17020516978313083, 54.91041666571061342, -6.403925809002825709 ) ) ;
#6340=EDGE_CURVE ( 'NONE', #6740, #5854, #3788, .T. ) ;
#6346=CARTESIAN_POINT ( 'NONE',  ( -23.98076211353314235, 52.97083333142136752, -6.154700538379337615 ) ) ;
#6361=EDGE_CURVE ( 'NONE', #1944, #1390, #9012, .T. ) ;
#6372=CARTESIAN_POINT ( 'NONE',  ( -24.98076211353313170, 53.49583333142136610, -3.267949192431250705 ) ) ;
#6374=CARTESIAN_POINT ( 'NONE',  ( -24.35964822603314772, 52.75208333237727487, -5.935950539335252074 ) ) ;
#6380=ADVANCED_FACE ( 'NONE', ( #6665 ), #10064, .F. ) ;
#6381=ORIENTED_EDGE ( 'NONE', *, *, #4243, .T. ) ;
#6382=CYLINDRICAL_SURFACE ( 'NONE', #4161, 1.999999999999971356 ) ;
#6383=CARTESIAN_POINT ( 'NONE',  ( -24.35964822603314772, 51.06041666571061910, -4.064049460664953983 ) ) ;
#6395=CARTESIAN_POINT ( 'NONE',  ( -23.98076211353314235, 52.21249999808803466, -5.000000000000103029 ) ) ;
#6397=CARTESIAN_POINT ( 'NONE',  ( -26.98076211353309972, 53.23333333333319217, -6.732050807568954909 ) ) ;
#6399=ORIENTED_EDGE ( 'NONE', *, *, #4243, .F. ) ;
#6401=CARTESIAN_POINT ( 'NONE',  ( -27.98076211353308551, 49.79166666666652930, -6.154700538379338504 ) ) ;
#6409=EDGE_CURVE ( 'NONE', #276, #2646, #9393, .T. ) ;
#6413=LINE ( 'NONE', #3246, #1859 ) ;
#6415=CARTESIAN_POINT ( 'NONE',  ( -25.98076211353311393, 51.77499999999986358, -7.000000000000072831 ) ) ;
#6416=CARTESIAN_POINT ( 'NONE',  ( -27.60187600103308014, 53.68541666571061199, -5.935950539335252074 ) ) ;
#6417=DIRECTION ( 'NONE',  ( 0.000000000000000000, 0.000000000000000000, 1.000000000000000000 ) ) ;
#6421=CARTESIAN_POINT ( 'NONE',  ( -23.98076211353314235, 54.37083333142137320, -6.154700538379337615 ) ) ;
#6425=CARTESIAN_POINT ( 'NONE',  ( -25.17020516978313083, 50.71041666571061057, -6.403925809002825709 ) ) ;
#6427=VECTOR ( 'NONE', #3614, 1000.000000000000000 ) ;
#6432=ORIENTED_EDGE ( 'NONE', *, *, #5699, .F. ) ;
#6441=CARTESIAN_POINT ( 'NONE',  ( -25.98076211353311393, 51.68749999808803608, -7.309401076758571314 ) ) ;
#6443=CARTESIAN_POINT ( 'NONE',  ( -27.98076211353308551, 51.10416666475469327, -6.154700538379338504 ) ) ;
#6445=ORIENTED_EDGE ( 'NONE', *, *, #2398, .T. ) ;
#6462=( BOUNDED_CURVE ( )  B_SPLINE_CURVE ( 1, ( #8279, #550 ),
 .UNSPECIFIED., .F., .F. ) 
 B_SPLINE_CURVE_WITH_KNOTS ( ( 2, 2 ),
 ( 0.000000000000000000, 1.000000000000000000 ),
 .UNSPECIFIED. ) 
 CURVE ( )  GEOMETRIC_REPRESENTATION_ITEM ( )  RATIONAL_B_SPLINE_CURVE ( ( 0.9343183816103359796, 0.9343183816103359796 ) ) 
 REPRESENTATION_ITEM ( '' )  );
#6468=CARTESIAN_POINT ( 'NONE',  ( -26.79131905728310059, 50.65208333237728766, -6.403925809002825709 ) ) ;
#6474=CARTESIAN_POINT ( 'NONE',  ( -25.98076211353310683, 54.13749999808803182, -3.000000000000132339 ) ) ;
#6477=CARTESIAN_POINT ( 'NONE',  ( -26.98076211353408382, 57.99999999999985789, -9.000000000000701661 ) ) ;
#6479=CARTESIAN_POINT ( 'NONE',  ( -27.60187600103308725, 54.91041666571061342, -5.935950539335252074 ) ) ;
#6481=CARTESIAN_POINT ( 'NONE',  ( -24.35964822603314772, 53.86041666571062336, -4.064049460664953983 ) ) ;
#6482=EDGE_LOOP ( 'NONE', ( #1212, #799, #6445, #10995 ) ) ;
#6490=AXIS2_PLACEMENT_3D ( 'NONE', #8469, #4255, #14 ) ;
#6491=ORIENTED_EDGE ( 'NONE', *, *, #7162, .T. ) ;
#6496=CARTESIAN_POINT ( 'NONE',  ( -24.98076211353313170, 53.49583333142136610, -3.267949192431250705 ) ) ;
#6503=CARTESIAN_POINT ( 'NONE',  ( -25.98076211353311393, 52.47499999999985931, -7.000000000000072831 ) ) ;
#6504=CIRCLE ( 'NONE', #656, 4.000000000000600409 ) ;
#6511=CARTESIAN_POINT ( 'NONE',  ( -25.98076211353311393, 51.33749999808802755, -3.000000000000132783 ) ) ;
#6512=VERTEX_POINT ( 'NONE', #2566 ) ;
#6515=CARTESIAN_POINT ( 'NONE',  ( -25.98076211353311038, 61.49999999999985789, -1.499999999999510392 ) ) ;
#6517=CARTESIAN_POINT ( 'NONE',  ( -23.98076211353314235, 52.27083333142136468, -6.154700538379337615 ) ) ;
#6520=CARTESIAN_POINT ( 'NONE',  ( -24.35964822603314772, 51.87708333237728908, -5.935950539335252074 ) ) ;
#6529=DIRECTION ( 'NONE',  ( 0.000000000000000000, 1.000000000000000000, 0.000000000000000000 ) ) ;
#6531=( BOUNDED_CURVE ( )  B_SPLINE_CURVE ( 2, ( #9553, #1099, #5122, #10224, #8500, #4505, #5173, #4337, #880 ),
 .UNSPECIFIED., .F., .F. ) 
 B_SPLINE_CURVE_WITH_KNOTS ( ( 3, 2, 2, 2, 3 ),
 ( 0.2500000000000000000, 0.2592592592592592449, 0.2777777777777777901, 0.2962962962962962798, 0.3055555555555555802 ),
 .UNSPECIFIED. ) 
 CURVE ( )  GEOMETRIC_REPRESENTATION_ITEM ( )  RATIONAL_B_SPLINE_CURVE ( ( 0.9330127018922192983, 0.9330127018922194093, 1.000000000000000000, 0.8660254037844387076, 1.000000000000000000, 0.8660254037844387076, 1.000000000000000000, 0.9330127018922191873, 0.9330127018922194093 ) ) 
 REPRESENTATION_ITEM ( '' )  );
#6532=EDGE_CURVE ( 'NONE', #5764, #10879, #6828, .T. ) ;
#6534=B_SPLINE_CURVE_WITH_KNOTS ( 'NONE', 3,
 ( #9691, #5475, #8909, #1925, #4640, #10583, #3693, #5312, #1073, #10417 ),
 .UNSPECIFIED., .F., .F.,
 ( 4, 2, 2, 2, 4 ),
 ( 0.003180982857628660964, 0.003578183968417414373, 0.003975385079206167349, 0.004372586189994920325, 0.004769787300783674168 ),
 .UNSPECIFIED. ) ;
#6535=CARTESIAN_POINT ( 'NONE',  ( -25.98076211353310683, 53.04374999904395338, -3.128098921329806714 ) ) ;
#6537=CARTESIAN_POINT ( 'NONE',  ( -23.98076211353314235, 50.14166666666653072, -3.845299461620867554 ) ) ;
#6539=CARTESIAN_POINT ( 'NONE',  ( -27.60187600103308370, 55.84374999904394343, -5.000000000000103029 ) ) ;
#6540=EDGE_CURVE ( 'NONE', #8562, #3014, #1387, .T. ) ;
#6553=CARTESIAN_POINT ( 'NONE',  ( -27.98076211353308551, 50.46249999808803466, -5.000000000000103029 ) ) ;
#6566=DIRECTION ( 'NONE',  ( 0.000000000000000000, 1.000000000000000000, 0.000000000000000000 ) ) ;
#6573=CARTESIAN_POINT ( 'NONE',  ( -25.98076211353311393, 50.59374999904395054, -6.871901078670400231 ) ) ;
#6578=DIRECTION ( 'NONE',  ( 1.000000000000000000, 0.000000000000000000, 0.000000000000000000 ) ) ;
#6579=CARTESIAN_POINT ( 'NONE',  ( -26.79131905728310059, 50.82708333237727771, -6.403925809002825709 ) ) ;
#6580=CARTESIAN_POINT ( 'NONE',  ( -26.79131905728310059, 52.05208333237728624, -6.403925809002825709 ) ) ;
#6582=CARTESIAN_POINT ( 'NONE',  ( -23.98076211353314235, 51.59999999999985931, -5.000000000000103029 ) ) ;
#6586=ORIENTED_EDGE ( 'NONE', *, *, #7144, .F. ) ;
#6600=CARTESIAN_POINT ( 'NONE',  ( -27.98076211353308551, 52.62083333142137320, -3.845299461620869330 ) ) ;
#6601=CARTESIAN_POINT ( 'NONE',  ( -25.98076211353311393, 53.17499999999985505, -7.000000000000072831 ) ) ;
#6603=EDGE_LOOP ( 'NONE', ( #4215, #7834, #9094, #10352 ) ) ;
#6608=CARTESIAN_POINT ( 'NONE',  ( -25.98076211353311393, 52.12499999999985079, -3.000000000000132339 ) ) ;
#6610=CARTESIAN_POINT ( 'NONE',  ( -26.95376948895698987, 57.73464630110304796, -3.251713298125628704 ) ) ;
#6614=CARTESIAN_POINT ( 'NONE',  ( -26.51666049839535688, 55.21876073720499534, -7.000000000000071942 ) ) ;
#6620=CARTESIAN_POINT ( 'NONE',  ( -25.98076211353311393, 54.83749999808802755, -3.000000000000132339 ) ) ;
#6624=CARTESIAN_POINT ( 'NONE',  ( -25.17020516978313083, 49.83541666571061768, -6.403925809002825709 ) ) ;
#6625=AXIS2_PLACEMENT_3D ( 'NONE', #6036, #1705, #10923 ) ;
#6628=DIRECTION ( 'NONE',  ( 0.000000000000000000, -1.000000000000000000, 0.000000000000000000 ) ) ;
#6637=CARTESIAN_POINT ( 'NONE',  ( -25.98076211353310683, 51.64374999904395480, -3.128098921329806714 ) ) ;
#6641=CARTESIAN_POINT ( 'NONE',  ( -23.98076211353314235, 52.35833333333319928, -6.154700538379337615 ) ) ;
#6644=VERTEX_POINT ( 'NONE', #2851 ) ;
#6645=ORIENTED_EDGE ( 'NONE', *, *, #2417, .F. ) ;
#6646=ORIENTED_EDGE ( 'NONE', *, *, #10826, .T. ) ;
#6658=CARTESIAN_POINT ( 'NONE',  ( -24.35964822603314772, 50.65208333237728056, -5.935950539335252074 ) ) ;
#6661=CARTESIAN_POINT ( 'NONE',  ( -25.98076211353311393, 55.18749999808802897, -7.309401076758571314 ) ) ;
#6665=FACE_OUTER_BOUND ( 'NONE', #4555, .T. ) ;
#6674=AXIS2_PLACEMENT_3D ( 'NONE', #5869, #10262, #9307 ) ;
#6675=CARTESIAN_POINT ( 'NONE',  ( -25.36399665479294896, 58.79766018380388459, -6.905020239873124410 ) ) ;
#6677=CARTESIAN_POINT ( 'NONE',  ( -26.98076211353408027, 57.86781137917856910, -3.267949192431818251 ) ) ;
#6685=CARTESIAN_POINT ( 'NONE',  ( -25.98076211353311393, 51.77499999999986358, -7.000000000000072831 ) ) ;
#6693=CARTESIAN_POINT ( 'NONE',  ( -24.35964822603314772, 55.43541666571061199, -4.064049460664953983 ) ) ;
#6695=LINE ( 'NONE', #1813, #1398 ) ;
#6701=CARTESIAN_POINT ( 'NONE',  ( -27.60187600103308370, 53.74374999904394201, -5.000000000000103029 ) ) ;
#6702=CARTESIAN_POINT ( 'NONE',  ( -25.98076211353310683, 52.69374999904395196, -6.871901078670399343 ) ) ;
#6707=CARTESIAN_POINT ( 'NONE',  ( -24.98076211353312814, 53.11666666666652503, -6.732050807568954909 ) ) ;
#6711=ORIENTED_EDGE ( 'NONE', *, *, #8671, .F. ) ;
#6714=ORIENTED_EDGE ( 'NONE', *, *, #2398, .F. ) ;
#6724=CARTESIAN_POINT ( 'NONE',  ( -24.98076211353312814, 54.42916666475469611, -6.732050807568954909 ) ) ;
#6727=CARTESIAN_POINT ( 'NONE',  ( -26.98076211353309972, 50.34583333142136752, -6.732050807568954909 ) ) ;
#6734=CARTESIAN_POINT ( 'NONE',  ( -26.24738432486657302, 57.02739972993323647, -3.014058635233636707 ) ) ;
#6736=CARTESIAN_POINT ( 'NONE',  ( -24.98076211353312814, 51.62916666475469896, -6.732050807568954909 ) ) ;
#6738=DIRECTION ( 'NONE',  ( 0.000000000000000000, 0.000000000000000000, 1.000000000000000000 ) ) ;
#6740=VERTEX_POINT ( 'NONE', #4512 ) ;
#6742=CARTESIAN_POINT ( 'NONE',  ( -27.98076211353308551, 54.60416666475470038, -6.154700538379338504 ) ) ;
#6746=DIRECTION ( 'NONE',  ( 0.000000000000000000, 0.000000000000000000, 1.000000000000000000 ) ) ;
#6747=CARTESIAN_POINT ( 'NONE',  ( -25.98076211353311393, 54.44374999904394485, -3.128098921329806714 ) ) ;
#6750=CARTESIAN_POINT ( 'NONE',  ( -25.84608536423723635, 56.99999999999889866, -3.000000000000131450 ) ) ;
#6754=CARTESIAN_POINT ( 'NONE',  ( -27.98076211353308551, 53.32083333142136894, -3.845299461620869330 ) ) ;
#6755=CARTESIAN_POINT ( 'NONE',  ( -25.17020516978313083, 53.27708333237728056, -3.596074190997380349 ) ) ;
#6759=CARTESIAN_POINT ( 'NONE',  ( -23.98076211353314235, 50.84166666666652645, -3.845299461620867554 ) ) ;
#6761=ORIENTED_EDGE ( 'NONE', *, *, #10105, .F. ) ;
#6764=ORIENTED_EDGE ( 'NONE', *, *, #5137, .F. ) ;
#6772=CARTESIAN_POINT ( 'NONE',  ( -25.98076211353311393, 49.49999999999986500, -7.000000000000074607 ) ) ;
#6776=CARTESIAN_POINT ( 'NONE',  ( -25.98076211353311393, 51.11874999904394201, -3.128098921329806714 ) ) ;
#6779=CARTESIAN_POINT ( 'NONE',  ( -25.98076211353311393, 49.49999999999986500, -7.000000000000074607 ) ) ;
#6780=PRODUCT_DEFINITION_SHAPE ( 'NONE', 'NONE',  #8571 ) ;
#6788=CARTESIAN_POINT ( 'NONE',  ( -24.35964822603314772, 52.57708333237728482, -5.935950539335252074 ) ) ;
#6801=CARTESIAN_POINT ( 'NONE',  ( -24.35964822603314417, 52.51874999904394770, -5.000000000000103029 ) ) ;
#6808=CARTESIAN_POINT ( 'NONE',  ( -27.60187600103308370, 54.44374999904394485, -5.000000000000103029 ) ) ;
#6813=CARTESIAN_POINT ( 'NONE',  ( -24.98076211353313170, 53.58333333333320070, -3.267949192431250705 ) ) ;
#6817=VERTEX_POINT ( 'NONE', #8163 ) ;
#6824=DIRECTION ( 'NONE',  ( 0.000000000000000000, 0.000000000000000000, 1.000000000000000000 ) ) ;
#6828=( BOUNDED_CURVE ( )  B_SPLINE_CURVE ( 2, ( #5950, #4172, #6727, #5072, #2507, #5894, #9279, #5181, #8508 ),
 .UNSPECIFIED., .F., .F. ) 
 B_SPLINE_CURVE_WITH_KNOTS ( ( 3, 2, 2, 2, 3 ),
 ( 0.02777777777777777971, 0.03703703703703703498, 0.05555555555555555247, 0.07407407407407406996, 0.08333333333333338422 ),
 .UNSPECIFIED. ) 
 CURVE ( )  GEOMETRIC_REPRESENTATION_ITEM ( )  RATIONAL_B_SPLINE_CURVE ( ( 0.9330127018922194093, 0.9330127018922194093, 1.000000000000000000, 0.8660254037844387076, 1.000000000000000000, 0.8660254037844387076, 1.000000000000000000, 0.9330127018922189652, 0.9330127018922194093 ) ) 
 REPRESENTATION_ITEM ( '' )  );
#6830=CARTESIAN_POINT ( 'NONE',  ( -27.60187600103308370, 50.24374999904394912, -5.000000000000103029 ) ) ;
#6835=CARTESIAN_POINT ( 'NONE',  ( -24.35964822603314772, 50.53541666571060631, -4.064049460664953983 ) ) ;
#6837=CARTESIAN_POINT ( 'NONE',  ( -25.98076211353310683, 53.52499999999986358, -3.000000000000132339 ) ) ;
#6839=CARTESIAN_POINT ( 'NONE',  ( -25.36463575557657180, 58.79801918157050977, -3.094798637517150564 ) ) ;
#6846=CARTESIAN_POINT ( 'NONE',  ( -25.10866622795798619, 58.50632701280146364, -6.800737734245783095 ) ) ;
#6849=CARTESIAN_POINT ( 'NONE',  ( -24.35964822603314772, 52.46041666571062478, -4.064049460664953983 ) ) ;
#6852=CARTESIAN_POINT ( 'NONE',  ( -26.77852525657794658, 58.61651288262306281, -6.836577306127424869 ) ) ;
#6862=CARTESIAN_POINT ( 'NONE',  ( -27.60187600103308014, 52.22708333237728340, -4.064049460664955760 ) ) ;
#6866=ORIENTED_EDGE ( 'NONE', *, *, #2787, .T. ) ;
#6868=ADVANCED_FACE ( 'NONE', ( #1490 ), #7021, .T. ) ;
#6871=CARTESIAN_POINT ( 'NONE',  ( -26.79131905728310059, 52.92708333237727913, -6.403925809002825709 ) ) ;
#6872=CARTESIAN_POINT ( 'NONE',  ( -23.98076211353314235, 50.89999999999986358, -5.000000000000103029 ) ) ;
#6877=CARTESIAN_POINT ( 'NONE',  ( -25.98076211353311393, 54.92499999999986926, -2.690598923241634743 ) ) ;
#6893=CARTESIAN_POINT ( 'NONE',  ( -24.35964822603314417, 54.09374999904395054, -5.000000000000103029 ) ) ;
#6895=ADVANCED_FACE ( 'NONE', ( #5561 ), #8942, .T. ) ;
#6899=CARTESIAN_POINT ( 'NONE',  ( -25.98076211353311393, 54.83749999808803466, -2.690598923241634743 ) ) ;
#6901=CARTESIAN_POINT ( 'NONE',  ( -25.44486372867087809, 53.84373926088289863, -7.000000000000075495 ) ) ;
#6906=ORIENTED_EDGE ( 'NONE', *, *, #9474, .T. ) ;
#6910=CARTESIAN_POINT ( 'NONE',  ( -24.35964822603314772, 49.77708333237728766, -5.935950539335252074 ) ) ;
#6913=CARTESIAN_POINT ( 'NONE',  ( -25.98076211353311393, 51.42499999999986926, -3.000000000000132783 ) ) ;
#6919=CARTESIAN_POINT ( 'NONE',  ( -25.98076211353311038, 57.99999999999985789, -9.000000000000701661 ) ) ;
#6921=CARTESIAN_POINT ( 'NONE',  ( -25.98076211353311393, 51.99374999904394912, -6.871901078670400231 ) ) ;
#6930=CARTESIAN_POINT ( 'NONE',  ( -25.17020516978313083, 54.67708333237727913, -3.596074190997380349 ) ) ;
#6931=CARTESIAN_POINT ( 'NONE',  ( -25.98076211353310683, 54.92499999999986926, -3.000000000000132339 ) ) ;
#6932=DIRECTION ( 'NONE',  ( 0.000000000000000000, 1.000000000000000000, 0.000000000000000000 ) ) ;
#6946=CARTESIAN_POINT ( 'NONE',  ( -24.35964822603314417, 53.39374999904394770, -5.000000000000103029 ) ) ;
#6956=CARTESIAN_POINT ( 'NONE',  ( 0.000000000000000000, 0.000000000000000000, 0.000000000000000000 ) ) ;
#6960=CARTESIAN_POINT ( 'NONE',  ( -25.17020516978313083, 49.83541666571061768, -6.403925809002825709 ) ) ;
#6965=ORIENTED_EDGE ( 'NONE', *, *, #1042, .F. ) ;
#6974=CARTESIAN_POINT ( 'NONE',  ( -27.60187600103308014, 55.61041666571061626, -5.935950539335252074 ) ) ;
#6976=( NAMED_UNIT ( * ) PLANE_ANGLE_UNIT ( ) SI_UNIT ( $, .RADIAN. ) );
#6977=CYLINDRICAL_SURFACE ( 'NONE', #2581, 1.999999999999971356 ) ;
#6983=UNCERTAINTY_MEASURE_WITH_UNIT (LENGTH_MEASURE( 1.000000000000000082E-05 ), #3841, 'distance_accuracy_value', 'NONE');
#6986=CARTESIAN_POINT ( 'NONE',  ( -24.98076211353312814, 55.21666666666653356, -6.732050807568954909 ) ) ;
#7001=CARTESIAN_POINT ( 'NONE',  ( -26.79131905728310059, 54.32708333237727771, -6.403925809002825709 ) ) ;
#7015=CARTESIAN_POINT ( 'NONE',  ( -24.35964822603314772, 51.87708333237728908, -5.935950539335252074 ) ) ;
#7021=CONICAL_SURFACE ( 'NONE', #10549, 3.500000000000591971, 0.7853981633974560506 ) ;
#7023=CARTESIAN_POINT ( 'NONE',  ( -25.98076211353311393, 53.08749999808803466, -7.000000000000072831 ) ) ;
#7031=VECTOR ( 'NONE', #3079, 1000.000000000000000 ) ;
#7035=CARTESIAN_POINT ( 'NONE',  ( -25.98076211353311393, 49.49999999999986500, -7.000000000000074607 ) ) ;
#7049=DIRECTION ( 'NONE',  ( 0.000000000000000000, 1.000000000000000000, 0.000000000000000000 ) ) ;
#7062=CARTESIAN_POINT ( 'NONE',  ( -25.17020516978313083, 53.97708333237728340, -3.596074190997380349 ) ) ;
#7066=PRODUCT ( 'Cable Pinch Bolt Clamp', 'Cable Pinch Bolt Clamp', '', ( #160 ) ) ;
#7072=SURFACE_SIDE_STYLE ('',( #7905 ) ) ;
#7076=CARTESIAN_POINT ( 'NONE',  ( -24.35964822603314772, 53.27708333237728056, -5.935950539335252074 ) ) ;
#7095=CARTESIAN_POINT ( 'NONE',  ( -23.98076211353314235, 55.07083333142136894, -6.154700538379337615 ) ) ;
#7099=CARTESIAN_POINT ( 'NONE',  ( -27.60187600103308014, 54.38541666571060773, -5.935950539335252074 ) ) ;
#7101=CARTESIAN_POINT ( 'NONE',  ( -25.98076211353311393, 54.57499999999985363, -7.309401076758571314 ) ) ;
#7107=CARTESIAN_POINT ( 'NONE',  ( -27.78269167149760577, 55.70378148983614608, -4.132215540378284757 ) ) ;
#7112=CARTESIAN_POINT ( 'NONE',  ( -24.35964822603314772, 54.15208333237728766, -5.935950539335252074 ) ) ;
#7122=CARTESIAN_POINT ( 'NONE',  ( -27.60187600103308370, 55.69181177612239253, -4.629976868092589903 ) ) ;
#7130=DIRECTION ( 'NONE',  ( 0.000000000000000000, 1.000000000000000000, 0.000000000000000000 ) ) ;
#7134=CARTESIAN_POINT ( 'NONE',  ( -27.44132332507749794, 55.71836679508493262, -4.296600267573891685 ) ) ;
#7139=CARTESIAN_POINT ( 'NONE',  ( -25.98076211353311038, 49.67499999999986215, -7.000000000000072831 ) ) ;
#7144=EDGE_CURVE ( 'NONE', #10879, #6740, #2349, .T. ) ;
#7148=CARTESIAN_POINT ( 'NONE',  ( -25.98076211353311393, 51.81874999904394485, -3.128098921329806714 ) ) ;
#7152=CARTESIAN_POINT ( 'NONE',  ( -25.98076211353311393, 49.49999999999986500, -5.000000000000103029 ) ) ;
#7161=CARTESIAN_POINT ( 'NONE',  ( -24.35964822603314772, 52.05208333237727913, -5.935950539335252074 ) ) ;
#7162=EDGE_CURVE ( 'NONE', #6093, #3608, #6051, .T. ) ;
#7163=ORIENTED_EDGE ( 'NONE', *, *, #5137, .T. ) ;
#7165=ORIENTED_EDGE ( 'NONE', *, *, #4850, .T. ) ;
#7176=CARTESIAN_POINT ( 'NONE',  ( -23.98076211353314235, 50.17083333142137036, -6.154700538379337615 ) ) ;
#7177=CARTESIAN_POINT ( 'NONE',  ( -23.98076211353314235, 52.85416666475470038, -3.845299461620867554 ) ) ;
#7180=ORIENTED_EDGE ( 'NONE', *, *, #4683, .F. ) ;
#7185=CARTESIAN_POINT ( 'NONE',  ( -25.98076211353311038, 49.67499999999986215, -7.000000000000072831 ) ) ;
#7186=( BOUNDED_CURVE ( )  B_SPLINE_CURVE ( 2, ( #8310, #9422, #2661, #9305, #4939, #1647, #10984, #5979, #8417 ),
 .UNSPECIFIED., .F., .F. ) 
 B_SPLINE_CURVE_WITH_KNOTS ( ( 3, 2, 2, 2, 3 ),
 ( 0.1388888888888888951, 0.1481481481481481399, 0.1666666666666666574, 0.1851851851851851749, 0.1944444444444444475 ),
 .UNSPECIFIED. ) 
 CURVE ( )  GEOMETRIC_REPRESENTATION_ITEM ( )  RATIONAL_B_SPLINE_CURVE ( ( 0.9330127018922192983, 0.9330127018922194093, 1.000000000000000000, 0.8660254037844387076, 1.000000000000000000, 0.8660254037844387076, 1.000000000000000000, 0.9330127018922191873, 0.9330127018922192983 ) ) 
 REPRESENTATION_ITEM ( '' )  );
#7193=CARTESIAN_POINT ( 'NONE',  ( -25.98076211353311393, 49.49999999999986500, -7.000000000000074607 ) ) ;
#7202=CARTESIAN_POINT ( 'NONE',  ( -26.51666049839535333, 51.39373926088290290, -3.000000000000132339 ) ) ;
#7203=CARTESIAN_POINT ( 'NONE',  ( -26.79131905728310059, 51.76041666571061484, -3.596074190997381237 ) ) ;
#7205=CARTESIAN_POINT ( 'NONE',  ( -27.98076211353308551, 55.44999999999986073, -5.000000000000103029 ) ) ;
#7214=CARTESIAN_POINT ( 'NONE',  ( -27.60187600103308370, 50.06874999904395196, -5.000000000000103029 ) ) ;
#7226=ADVANCED_FACE ( 'NONE', ( #3770 ), #1887, .T. ) ;
#7242=CARTESIAN_POINT ( 'NONE',  ( -25.84741345379021737, 56.99999999999889155, -7.000000000000078160 ) ) ;
#7251=CARTESIAN_POINT ( 'NONE',  ( -25.98076211353311393, 49.49999999999986500, -5.000000000000103029 ) ) ;
#7254=CARTESIAN_POINT ( 'NONE',  ( -25.44486372867087809, 53.46876073720499534, -3.000000000000132339 ) ) ;
#7256=CARTESIAN_POINT ( 'NONE',  ( -25.98076211353311393, 53.56874999904394485, -6.871901078670400231 ) ) ;
#7266=CARTESIAN_POINT ( 'NONE',  ( -27.60187600103308725, 50.82708333237729192, -4.064049460664955760 ) ) ;
#7280=CARTESIAN_POINT ( 'NONE',  ( -23.98076211353314235, 50.75416666475469185, -3.845299461620867554 ) ) ;
#7297=ADVANCED_FACE ( 'NONE', ( #7370 ), #7422, .F. ) ;
#7298=ORIENTED_EDGE ( 'NONE', *, *, #5536, .T. ) ;
#7306=CARTESIAN_POINT ( 'NONE',  ( -25.17020516978313083, 50.53541666571062052, -6.403925809002825709 ) ) ;
#7308=CARTESIAN_POINT ( 'NONE',  ( -26.98076211353309972, 55.33333333333320070, -6.732050807568954909 ) ) ;
#7314=EDGE_CURVE ( 'NONE', #9083, #7830, #2928, .T. ) ;
#7315=CARTESIAN_POINT ( 'NONE',  ( -24.35964822603314772, 50.53541666571060631, -4.064049460664953983 ) ) ;
#7316=CARTESIAN_POINT ( 'NONE',  ( -27.60187600103308370, 53.56874999904395196, -5.000000000000103029 ) ) ;
#7317=AXIS2_PLACEMENT_3D ( 'NONE', #4508, #9389, #10390 ) ;
#7319=CARTESIAN_POINT ( 'NONE',  ( -26.79131905728310059, 54.38541666571061484, -3.596074190997381237 ) ) ;
#7332=CARTESIAN_POINT ( 'NONE',  ( -25.98076211353311393, 51.33749999808802755, -2.690598923241634743 ) ) ;
#7346=DIRECTION ( 'NONE',  ( 0.000000000000000000, 1.000000000000000000, 0.000000000000000000 ) ) ;
#7349=CARTESIAN_POINT ( 'NONE',  ( -26.51666049839534622, 55.50623925897107114, -3.000000000000131006 ) ) ;
#7350=ADVANCED_FACE ( 'NONE', ( #4775 ), #1430, .T. ) ;
#7358=ADVANCED_FACE ( 'NONE', ( #3878 ), #4035, .T. ) ;
#7360=CARTESIAN_POINT ( 'NONE',  ( -27.60187600103308014, 50.12708333237727487, -4.064049460664955760 ) ) ;
#7362=LINE ( 'NONE', #525, #4310 ) ;
#7363=CARTESIAN_POINT ( 'NONE',  ( -25.98076211353311393, 55.27499999999985647, -7.000000000000072831 ) ) ;
#7365=ORIENTED_EDGE ( 'NONE', *, *, #9983, .T. ) ;
#7366=( BOUNDED_CURVE ( )  B_SPLINE_CURVE ( 2, ( #4591, #4532, #9633, #511, #10684, #3694, #2025, #5418, #3747 ),
 .UNSPECIFIED., .F., .F. ) 
 B_SPLINE_CURVE_WITH_KNOTS ( ( 3, 2, 2, 2, 3 ),
 ( 0.3611111111111111605, 0.3703703703703703498, 0.3888888888888888951, 0.4074074074074073848, 0.4166666666666666852 ),
 .UNSPECIFIED. ) 
 CURVE ( )  GEOMETRIC_REPRESENTATION_ITEM ( )  RATIONAL_B_SPLINE_CURVE ( ( 0.9330127018922194093, 0.9330127018922197424, 1.000000000000000000, 0.8660254037844387076, 1.000000000000000000, 0.8660254037844387076, 1.000000000000000000, 0.9330127018922191873, 0.9330127018922194093 ) ) 
 REPRESENTATION_ITEM ( '' )  );
#7370=FACE_OUTER_BOUND ( 'NONE', #9261, .T. ) ;
#7371=CARTESIAN_POINT ( 'NONE',  ( -26.79131905728310059, 50.36041666571060915, -3.596074190997381237 ) ) ;
#7373=CARTESIAN_POINT ( 'NONE',  ( -27.60187600103308370, 52.16874999904395338, -5.000000000000103029 ) ) ;
#7376=CARTESIAN_POINT ( 'NONE',  ( -25.17020516978313083, 54.50208333237728198, -3.596074190997380349 ) ) ;
#7389=CARTESIAN_POINT ( 'NONE',  ( -27.98076211353308551, 51.86249999808803324, -5.000000000000103029 ) ) ;
#7397=CARTESIAN_POINT ( 'NONE',  ( -23.98076211353314235, 52.35833333333319217, -6.154700538379337615 ) ) ;
#7406=ORIENTED_EDGE ( 'NONE', *, *, #3231, .T. ) ;
#7414=CARTESIAN_POINT ( 'NONE',  ( -25.98076211353311393, 52.82499999999986784, -3.000000000000132339 ) ) ;
#7415=CARTESIAN_POINT ( 'NONE',  ( -24.35964822603314772, 50.47708333237728340, -5.935950539335252074 ) ) ;
#7422=CYLINDRICAL_SURFACE ( 'NONE', #68, 1.000000000000972333 ) ;
#7425=CARTESIAN_POINT ( 'NONE',  ( -24.98076211353193798, 57.99999999999910472, -3.267949192431741423 ) ) ;
#7426=CARTESIAN_POINT ( 'NONE',  ( -24.35964822603314417, 52.51874999904394770, -5.000000000000103029 ) ) ;
#7428=CARTESIAN_POINT ( 'NONE',  ( -24.35964822603314772, 54.67708333237728624, -5.935950539335252074 ) ) ;
#7432=ORIENTED_EDGE ( 'NONE', *, *, #8873, .T. ) ;
#7443=EDGE_CURVE ( 'NONE', #10877, #8683, #7186, .T. ) ;
#7445=CARTESIAN_POINT ( 'NONE',  ( -27.98076211353308551, 51.10416666475470748, -6.154700538379338504 ) ) ;
#7457=CARTESIAN_POINT ( 'NONE',  ( -25.98076211353311393, 49.49999999999986500, -7.000000000000074607 ) ) ;
#7464=CARTESIAN_POINT ( 'NONE',  ( -27.98076211353308551, 51.94999999999986784, -5.000000000000103029 ) ) ;
#7467=CARTESIAN_POINT ( 'NONE',  ( -23.98076211353314235, 52.21249999808803466, -5.000000000000103029 ) ) ;
#7468=CARTESIAN_POINT ( 'NONE',  ( -27.78269984933782411, 56.11211482050296695, -4.132232521764788835 ) ) ;
#7470=CARTESIAN_POINT ( 'NONE',  ( -24.35964822603314772, 54.85208333237728340, -5.935950539335252074 ) ) ;
#7477=ADVANCED_FACE ( 'NONE', ( #10150 ), #800, .T. ) ;
#7480=CARTESIAN_POINT ( 'NONE',  ( -26.79131905728310059, 51.52708333237728056, -6.403925809002825709 ) ) ;
#7481=CARTESIAN_POINT ( 'NONE',  ( -25.17020516978313083, 53.80208333237728624, -3.596074190997380349 ) ) ;
#7483=CARTESIAN_POINT ( 'NONE',  ( -25.98076211353311393, 52.82499999999986784, -2.690598923241634743 ) ) ;
#7501=CARTESIAN_POINT ( 'NONE',  ( -27.98076211353308551, 56.08556146700746581, -4.543501304393035234 ) ) ;
#7503=DIRECTION ( 'NONE',  ( 2.775557561562891351E-17, 1.000000000000000000, -8.326672684688671588E-17 ) ) ;
#7521=CARTESIAN_POINT ( 'NONE',  ( -27.98076211353308551, 54.72083333142136041, -3.845299461620869330 ) ) ;
#7527=CARTESIAN_POINT ( 'NONE',  ( -27.60187600103308370, 50.76874999904395480, -5.000000000000103029 ) ) ;
#7534=CARTESIAN_POINT ( 'NONE',  ( -27.98076211353308551, 53.99166666666652503, -6.154700538379338504 ) ) ;
#7536=DIRECTION ( 'NONE',  ( 2.775557561562891351E-17, 1.000000000000000000, -8.326672684688671588E-17 ) ) ;
#7537=CARTESIAN_POINT ( 'NONE',  ( -24.35964822603314772, 54.67708333237728624, -5.935950539335252074 ) ) ;
#7541=CARTESIAN_POINT ( 'NONE',  ( -23.98076211353314235, 51.65833333333319644, -6.154700538379337615 ) ) ;
#7557=DIRECTION ( 'NONE',  ( 0.000000000000000000, 1.000000000000000000, 0.000000000000000000 ) ) ;
#7560=CARTESIAN_POINT ( 'NONE',  ( -27.98076211353308551, 54.60416666475469327, -6.154700538379338504 ) ) ;
#7572=CARTESIAN_POINT ( 'NONE',  ( -26.77929575296436582, 57.38439079953180766, -3.163742677926416835 ) ) ;
#7581=CARTESIAN_POINT ( 'NONE',  ( -26.98076211353309972, 54.54583333142136325, -6.732050807568954909 ) ) ;
#7587=DIRECTION ( 'NONE',  ( -0.000000000000000000, -0.000000000000000000, 1.000000000000000000 ) ) ;
#7589=CARTESIAN_POINT ( 'NONE',  ( -24.35964822603314772, 53.16041666571062763, -4.064049460664953983 ) ) ;
#7597=CARTESIAN_POINT ( 'NONE',  ( -26.79131905728310059, 54.32708333237727771, -6.403925809002825709 ) ) ;
#7598=ADVANCED_FACE ( 'NONE', ( #9943 ), #5719, .T. ) ;
#7604=CARTESIAN_POINT ( 'NONE',  ( -25.98076211353311393, 53.52499999999986358, -2.690598923241634743 ) ) ;
#7616=( BOUNDED_CURVE ( )  B_SPLINE_CURVE ( 2, ( #8801, #8863, #1184, #4587, #9689, #2082, #6131, #9522, #4639 ),
 .UNSPECIFIED., .F., .F. ) 
 B_SPLINE_CURVE_WITH_KNOTS ( ( 3, 2, 2, 2, 3 ),
 ( 0.08333333333333331483, 0.09259259259259258745, 0.1111111111111111049, 0.1296296296296296224, 0.1388888888888888951 ),
 .UNSPECIFIED. ) 
 CURVE ( )  GEOMETRIC_REPRESENTATION_ITEM ( )  RATIONAL_B_SPLINE_CURVE ( ( 0.9330127018922192983, 0.9330127018922191873, 1.000000000000000000, 0.8660254037844387076, 1.000000000000000000, 0.8660254037844387076, 1.000000000000000000, 0.9330127018922191873, 0.9330127018922192983 ) ) 
 REPRESENTATION_ITEM ( '' )  );
#7620=CARTESIAN_POINT ( 'NONE',  ( -27.60187600103308014, 50.30208333237727913, -4.064049460664955760 ) ) ;
#7624=ORIENTED_EDGE ( 'NONE', *, *, #9983, .F. ) ;
#7631=CARTESIAN_POINT ( 'NONE',  ( -24.35964822603314417, 49.71874999904395054, -5.000000000000103029 ) ) ;
#7634=CARTESIAN_POINT ( 'NONE',  ( -25.98076211353310683, 55.53749999808803040, -3.000000000000132339 ) ) ;
#7645=CARTESIAN_POINT ( 'NONE',  ( -26.79131905728310059, 53.45208333237728482, -6.403925809002825709 ) ) ;
#7647=DIRECTION ( 'NONE',  ( 0.000000000000000000, 1.000000000000000000, 0.000000000000000000 ) ) ;
#7655=CARTESIAN_POINT ( 'NONE',  ( -24.35964822603314417, 54.79374999904394627, -5.000000000000103029 ) ) ;
#7656=CARTESIAN_POINT ( 'NONE',  ( -25.98076211353310683, 55.49374999904395622, -6.871901078670399343 ) ) ;
#7660=CARTESIAN_POINT ( 'NONE',  ( -23.98076211353314235, 50.89999999999986358, -5.000000000000103029 ) ) ;
#7664=ORIENTED_EDGE ( 'NONE', *, *, #4025, .T. ) ;
#7667=ORIENTED_EDGE ( 'NONE', *, *, #1546, .F. ) ;
#7668=( BOUNDED_CURVE ( )  B_SPLINE_CURVE ( 2, ( #3749, #5315, #1251, #2924, #4643 ),
 .UNSPECIFIED., .F., .F. ) 
 B_SPLINE_CURVE_WITH_KNOTS ( ( 3, 2, 3 ),
 ( 0.000000000000000000, 0.01851851851851852096, 0.02777777777777775542 ),
 .UNSPECIFIED. ) 
 CURVE ( )  GEOMETRIC_REPRESENTATION_ITEM ( )  RATIONAL_B_SPLINE_CURVE ( ( 1.000000000000000000, 0.8660254037844387076, 1.000000000000000000, 0.9330127018922195203, 0.9330127018922194093 ) ) 
 REPRESENTATION_ITEM ( '' )  );
#7676=CARTESIAN_POINT ( 'NONE',  ( -25.98076211353311393, 55.88749999808803182, -7.309401076758571314 ) ) ;
#7689=CARTESIAN_POINT ( 'NONE',  ( -27.60187600103308370, 52.86874999904394912, -5.000000000000103029 ) ) ;
#7697=CARTESIAN_POINT ( 'NONE',  ( -26.98076211353309972, 51.83333333333319359, -6.732050807568954909 ) ) ;
#7699=CARTESIAN_POINT ( 'NONE',  ( -25.98076211353311393, 55.88749999808803182, -7.000000000000072831 ) ) ;
#7701=CARTESIAN_POINT ( 'NONE',  ( -24.35964822603314417, 55.31874999904395196, -5.000000000000103029 ) ) ;
#7709=CARTESIAN_POINT ( 'NONE',  ( -25.98076211353311393, 53.87499999999986500, -7.000000000000072831 ) ) ;
#7710=CARTESIAN_POINT ( 'NONE',  ( -25.98076211353310683, 52.86874999904393491, -6.871901078670399343 ) ) ;
#7712=CARTESIAN_POINT ( 'NONE',  ( -25.98076211353311393, 50.72499999999985931, -3.000000000000132783 ) ) ;
#7728=CARTESIAN_POINT ( 'NONE',  ( -24.35964822603314417, 50.59374999904394343, -5.000000000000103029 ) ) ;
#7731=CARTESIAN_POINT ( 'NONE',  ( -26.79131905728310059, 50.82708333237727771, -6.403925809002825709 ) ) ;
#7735=CARTESIAN_POINT ( 'NONE',  ( -25.71445732839318765, 58.97263009590939475, -3.014038965319806973 ) ) ;
#7736=ORIENTED_EDGE ( 'NONE', *, *, #10223, .T. ) ;
#7743=VECTOR ( 'NONE', #10125, 1000.000000000000000 ) ;
#7745=CARTESIAN_POINT ( 'NONE',  ( -25.98076211353311038, 61.49999999999985789, -0.9999999999995021760 ) ) ;
#7747=CARTESIAN_POINT ( 'NONE',  ( -26.79131905728310059, 50.88541666571061484, -3.596074190997381237 ) ) ;
#7752=EDGE_LOOP ( 'NONE', ( #5898, #8495, #7762, #3344 ) ) ;
#7756=CARTESIAN_POINT ( 'NONE',  ( -27.98076211353308551, 52.70833333333320780, -3.845299461620869330 ) ) ;
#7758=CARTESIAN_POINT ( 'NONE',  ( -24.35964822603314772, 53.86041666571062336, -4.064049460664953983 ) ) ;
#7762=ORIENTED_EDGE ( 'NONE', *, *, #4046, .F. ) ;
#7770=CARTESIAN_POINT ( 'NONE',  ( -25.17020516978313083, 54.21041666571061057, -6.403925809002825709 ) ) ;
#7776=CARTESIAN_POINT ( 'NONE',  ( -24.98076211353313170, 54.98333333333319928, -3.267949192431250705 ) ) ;
#7787=CARTESIAN_POINT ( 'NONE',  ( -25.98076211353311393, 54.22499999999985931, -3.000000000000132339 ) ) ;
#7791=FACE_OUTER_BOUND ( 'NONE', #8336, .T. ) ;
#7792=CARTESIAN_POINT ( 'NONE',  ( -25.98076211353311393, 53.56874999904394485, -6.871901078670400231 ) ) ;
#7795=ORIENTED_EDGE ( 'NONE', *, *, #10155, .F. ) ;
#7805=CARTESIAN_POINT ( 'NONE',  ( -24.35964822603314417, 52.51874999904394770, -5.000000000000103029 ) ) ;
#7809=VERTEX_POINT ( 'NONE', #10216 ) ;
#7813=CYLINDRICAL_SURFACE ( 'NONE', #1364, 1.999999999999971356 ) ;
#7815=CARTESIAN_POINT ( 'NONE',  ( -27.98076211353308551, 52.64999999999986358, -5.000000000000103029 ) ) ;
#7817=CARTESIAN_POINT ( 'NONE',  ( -24.35964822603314772, 55.37708333237728198, -5.935950539335252074 ) ) ;
#7818=PRESENTATION_STYLE_ASSIGNMENT (( #10478 ) ) ;
#7825=CARTESIAN_POINT ( 'NONE',  ( -23.98076211353314235, 55.09999999999986642, -5.000000000000103029 ) ) ;
#7830=VERTEX_POINT ( 'NONE', #3327 ) ;
#7834=ORIENTED_EDGE ( 'NONE', *, *, #6340, .T. ) ;
#7842=CARTESIAN_POINT ( 'NONE',  ( -25.98076211353311393, 53.91874999904394627, -3.128098921329806714 ) ) ;
#7854=CARTESIAN_POINT ( 'NONE',  ( -27.60187600103308014, 51.52708333237728766, -4.064049460664955760 ) ) ;
#7873=ORIENTED_EDGE ( 'NONE', *, *, #4731, .T. ) ;
#7882=CYLINDRICAL_SURFACE ( 'NONE', #1988, 1.999999999999971356 ) ;
#7895=CARTESIAN_POINT ( 'NONE',  ( -27.60187600103308014, 54.38541666571060773, -5.935950539335252074 ) ) ;
#7905=SURFACE_STYLE_FILL_AREA ( #8947 ) ;
#7909=CARTESIAN_POINT ( 'NONE',  ( -24.35964822603314417, 55.31874999904395196, -5.000000000000103029 ) ) ;
#7934=CARTESIAN_POINT ( 'NONE',  ( -26.77982134005685211, 57.38520624385693480, -6.835996254967358965 ) ) ;
#7935=CARTESIAN_POINT ( 'NONE',  ( -25.17020516978313083, 54.21041666571061057, -6.403925809002825709 ) ) ;
#7941=CARTESIAN_POINT ( 'NONE',  ( -27.98076211353308551, 54.80833333333319501, -3.845299461620869330 ) ) ;
#7947=AXIS2_PLACEMENT_3D ( 'NONE', #3185, #6566, #6738 ) ;
#7951=CARTESIAN_POINT ( 'NONE',  ( -25.17020516978313083, 51.87708333237728198, -3.596074190997380349 ) ) ;
#7962=CARTESIAN_POINT ( 'NONE',  ( -26.79131905728310059, 54.15208333237728056, -6.403925809002825709 ) ) ;
#7966=CARTESIAN_POINT ( 'NONE',  ( -24.98076211353312814, 53.02916666475469754, -6.732050807568954909 ) ) ;
#7971=FACE_OUTER_BOUND ( 'NONE', #958, .T. ) ;
#7974=CARTESIAN_POINT ( 'NONE',  ( -26.51666049839534267, 55.91876073720499818, -7.000000000000075495 ) ) ;
#7977=EDGE_CURVE ( 'NONE', #2292, #491, #5331, .T. ) ;
#7987=CARTESIAN_POINT ( 'NONE',  ( -25.44486372867087809, 55.15623925897106261, -7.000000000000075495 ) ) ;
#7989=ADVANCED_FACE ( 'NONE', ( #8766 ), #8830, .T. ) ;
#7991=CARTESIAN_POINT ( 'NONE',  ( -26.79131905728310059, 50.82708333237727771, -6.403925809002825709 ) ) ;
#7994=EDGE_LOOP ( 'NONE', ( #3056, #9559, #7165, #10768, #6761, #9669, #3342, #3768, #4178, #6711, #404, #6285, #8166, #9147 ) ) ;
#7996=CARTESIAN_POINT ( 'NONE',  ( -25.44486372867087454, 50.66876073720499818, -3.000000000000134559 ) ) ;
#7997=ADVANCED_FACE ( 'NONE', ( #9653 ), #4614, .T. ) ;
#8001=ORIENTED_EDGE ( 'NONE', *, *, #4731, .F. ) ;
#8003=CARTESIAN_POINT ( 'NONE',  ( -26.79131905728310059, 50.88541666571061484, -3.596074190997381237 ) ) ;
#8005=EDGE_LOOP ( 'NONE', ( #6098, #7873, #10601, #4292 ) ) ;
#8006=CARTESIAN_POINT ( 'NONE',  ( -25.17020516978313083, 53.51041666571060773, -6.403925809002825709 ) ) ;
#8007=ORIENTED_EDGE ( 'NONE', *, *, #8785, .T. ) ;
#8016=CARTESIAN_POINT ( 'NONE',  ( -23.98076211353314235, 49.55833333333319501, -6.154700538379337615 ) ) ;
#8039=CARTESIAN_POINT ( 'NONE',  ( -23.98076211353314235, 51.65833333333319644, -6.154700538379337615 ) ) ;
#8040=CARTESIAN_POINT ( 'NONE',  ( -27.60187600103308014, 51.00208333237728198, -4.064049460664955760 ) ) ;
#8069=EDGE_LOOP ( 'NONE', ( #9419, #8588, #6432, #6257 ) ) ;
#8071=ADVANCED_FACE ( 'NONE', ( #9366 ), #190, .T. ) ;
#8076=CARTESIAN_POINT ( 'NONE',  ( -27.98076211353308551, 56.06249999808802897, -5.000000000000103029 ) ) ;
#8082=FACE_OUTER_BOUND ( 'NONE', #6603, .T. ) ;
#8083=UNCERTAINTY_MEASURE_WITH_UNIT (LENGTH_MEASURE( 1.000000000000000082E-05 ), #4537, 'distance_accuracy_value', 'NONE');
#8087=( BOUNDED_CURVE ( )  B_SPLINE_CURVE ( 2, ( #6601, #4747, #6397, #4002, #4963, #3900, #10722, #9163, #3120 ),
 .UNSPECIFIED., .F., .F. ) 
 B_SPLINE_CURVE_WITH_KNOTS ( ( 3, 2, 2, 2, 3 ),
 ( 0.5833333333333333703, 0.5925925925925925597, 0.6111111111111111605, 0.6296296296296296502, 0.6388888888888889506 ),
 .UNSPECIFIED. ) 
 CURVE ( )  GEOMETRIC_REPRESENTATION_ITEM ( )  RATIONAL_B_SPLINE_CURVE ( ( 0.9330127018922194093, 0.9330127018922197424, 1.000000000000000000, 0.8660254037844387076, 1.000000000000000000, 0.8660254037844387076, 1.000000000000000000, 0.9330127018922189652, 0.9330127018922194093 ) ) 
 REPRESENTATION_ITEM ( '' )  );
#8093=CARTESIAN_POINT ( 'NONE',  ( -24.35964822603314772, 53.33541666571061057, -4.064049460664953983 ) ) ;
#8104=CARTESIAN_POINT ( 'NONE',  ( -25.17020516978313083, 51.23541666571061626, -6.403925809002825709 ) ) ;
#8108=CARTESIAN_POINT ( 'NONE',  ( -27.44132740410865523, 55.89336612041926600, -4.296608737464627126 ) ) ;
#8110=DIRECTION ( 'NONE',  ( 0.000000000000000000, 0.000000000000000000, 1.000000000000000000 ) ) ;
#8121=CARTESIAN_POINT ( 'NONE',  ( -26.98076211353309972, 51.04583333142137036, -6.732050807568954909 ) ) ;
#8147=CARTESIAN_POINT ( 'NONE',  ( -24.98076211353313170, 51.48333333333319928, -3.267949192431250705 ) ) ;
#8148=CARTESIAN_POINT ( 'NONE',  ( -27.60187600103308370, 50.94374999904394485, -5.000000000000103029 ) ) ;
#8153=CARTESIAN_POINT ( 'NONE',  ( -25.98076211353311393, 59.49999999999985789, -5.000000000000103029 ) ) ;
#8157=CARTESIAN_POINT ( 'NONE',  ( -25.17020516978313083, 51.93541666571061910, -6.403925809002825709 ) ) ;
#8161=CARTESIAN_POINT ( 'NONE',  ( -27.98076211353308551, 53.90416666475469754, -6.154700538379338504 ) ) ;
#8163=CARTESIAN_POINT ( 'NONE',  ( -27.44132332507749794, 55.71836679508493262, -4.296600267573891685 ) ) ;
#8166=ORIENTED_EDGE ( 'NONE', *, *, #8514, .T. ) ;
#8168=EDGE_CURVE ( 'NONE', #10992, #8562, #10492, .T. ) ;
#8172=CARTESIAN_POINT ( 'NONE',  ( -25.98076211353311393, 50.28749999808803040, -7.309401076758571314 ) ) ;
#8174=CARTESIAN_POINT ( 'NONE',  ( -25.98076211353311393, 50.98749999808804034, -7.000000000000073719 ) ) ;
#8178=ADVANCED_FACE ( 'NONE', ( #10199 ), #6977, .T. ) ;
#8186=LINE ( 'NONE', #7193, #7031 ) ;
#8196=CARTESIAN_POINT ( 'NONE',  ( -24.35964822603314772, 51.76041666571060773, -4.064049460664953983 ) ) ;
#8203=CARTESIAN_POINT ( 'NONE',  ( -25.98076211353311038, 59.49999999999985789, -5.000000000000102141 ) ) ;
#8204=CARTESIAN_POINT ( 'NONE',  ( -26.79131905728310059, 52.98541666571061626, -3.596074190997381237 ) ) ;
#8206=CARTESIAN_POINT ( 'NONE',  ( -26.79131905728310059, 55.55208333237728624, -6.403925809002825709 ) ) ;
#8209=ORIENTED_EDGE ( 'NONE', *, *, #3582, .F. ) ;
#8210=ORIENTED_EDGE ( 'NONE', *, *, #8514, .F. ) ;
#8218=CARTESIAN_POINT ( 'NONE',  ( -26.98076211353309972, 50.34583333142136752, -6.732050807568954909 ) ) ;
#8220=CARTESIAN_POINT ( 'NONE',  ( -25.98076211353311393, 51.33749999808802755, -3.000000000000132783 ) ) ;
#8238=EDGE_CURVE ( 'NONE', #4566, #5004, #4397, .T. ) ;
#8248=CARTESIAN_POINT ( 'NONE',  ( -24.35964822603314772, 55.55208333237727913, -5.935950539335252074 ) ) ;
#8254=AXIS2_PLACEMENT_3D ( 'NONE', #3370, #6628, #1644 ) ;
#8257=CARTESIAN_POINT ( 'NONE',  ( -25.17020516978313083, 50.47708333237727629, -3.596074190997380349 ) ) ;
#8259=CARTESIAN_POINT ( 'NONE',  ( -25.98076211353310683, 52.34374999904395054, -3.128098921329806714 ) ) ;
#8262=CARTESIAN_POINT ( 'NONE',  ( -27.98076211353308551, 49.79166666666652930, -6.154700538379338504 ) ) ;
#8264=CARTESIAN_POINT ( 'NONE',  ( -26.79131905728310059, 55.02708333237728056, -6.403925809002825709 ) ) ;
#8268=DIRECTION ( 'NONE',  ( 0.000000000000000000, -1.000000000000000000, 0.000000000000000000 ) ) ;
#8277=CARTESIAN_POINT ( 'NONE',  ( -23.98076211353314235, 50.11249999808803324, -5.000000000000103029 ) ) ;
#8279=CARTESIAN_POINT ( 'NONE',  ( -27.78268512908116961, 55.49961679590672503, -4.132201955500060642 ) ) ;
#8294=ORIENTED_EDGE ( 'NONE', *, *, #9732, .F. ) ;
#8297=CARTESIAN_POINT ( 'NONE',  ( -26.98076211353309972, 52.06666666666653498, -3.267949192431252037 ) ) ;
#8302=DIRECTION ( 'NONE',  ( 0.000000000000000000, 8.326672684688671588E-17, 1.000000000000000000 ) ) ;
#8303=CARTESIAN_POINT ( 'NONE',  ( -27.60187600103308014, 55.08541666571061057, -5.935950539335252074 ) ) ;
#8310=CARTESIAN_POINT ( 'NONE',  ( -25.98076211353311393, 50.37499999999987210, -7.000000000000073719 ) ) ;
#8311=CARTESIAN_POINT ( 'NONE',  ( -25.17020516978313083, 51.41041666571061342, -6.403925809002825709 ) ) ;
#8313=CARTESIAN_POINT ( 'NONE',  ( -26.79131905728310059, 53.45208333237728482, -6.403925809002825709 ) ) ;
#8315=( BOUNDED_CURVE ( )  B_SPLINE_CURVE ( 2, ( #3421, #5204, #6079, #1640, #5035, #4311, #9468, #792, #7699 ),
 .UNSPECIFIED., .F., .F. ) 
 B_SPLINE_CURVE_WITH_KNOTS ( ( 3, 2, 2, 2, 3 ),
 ( 0.8611111111111111605, 0.8703703703703703498, 0.8888888888888888395, 0.9074074074074074403, 0.9166666666666666297 ),
 .UNSPECIFIED. ) 
 CURVE ( )  GEOMETRIC_REPRESENTATION_ITEM ( )  RATIONAL_B_SPLINE_CURVE ( ( 0.9330127018922194093, 0.9330127018922197424, 1.000000000000000000, 0.8660254037844387076, 1.000000000000000000, 0.8660254037844387076, 1.000000000000000000, 0.9330127018922197424, 0.9330127018922194093 ) ) 
 REPRESENTATION_ITEM ( '' )  );
#8316=CARTESIAN_POINT ( 'NONE',  ( -24.98076211353313170, 51.48333333333319928, -3.267949192431250705 ) ) ;
#8332=CARTESIAN_POINT ( 'NONE',  ( -23.98076211353314235, 53.61249999808804034, -5.000000000000103029 ) ) ;
#8336=EDGE_LOOP ( 'NONE', ( #9889, #9625, #1961, #8812 ) ) ;
#8338=VERTEX_POINT ( 'NONE', #10168 ) ;
#8346=CARTESIAN_POINT ( 'NONE',  ( -23.98076211353314235, 51.45416666475470180, -3.845299461620867554 ) ) ;
#8350=ORIENTED_EDGE ( 'NONE', *, *, #1546, .T. ) ;
#8357=CARTESIAN_POINT ( 'NONE',  ( -27.60187600103308370, 50.06874999904395196, -5.000000000000103029 ) ) ;
#8365=CARTESIAN_POINT ( 'NONE',  ( -27.60187600103308370, 50.24374999904394912, -5.000000000000103029 ) ) ;
#8366=CARTESIAN_POINT ( 'NONE',  ( -25.17020516978313083, 54.50208333237728198, -3.596074190997380349 ) ) ;
#8368=CARTESIAN_POINT ( 'NONE',  ( -26.98076211353309972, 53.46666666666653356, -3.267949192431252037 ) ) ;
#8383=( BOUNDED_CURVE ( )  B_SPLINE_CURVE ( 2, ( #7787, #1047, #2619, #163, #3559, #2728, #6101, #9493, #4456 ),
 .UNSPECIFIED., .F., .F. ) 
 B_SPLINE_CURVE_WITH_KNOTS ( ( 3, 2, 2, 2, 3 ),
 ( 0.7500000000000000000, 0.7592592592592593004, 0.7777777777777777901, 0.7962962962962962798, 0.8055555555555555802 ),
 .UNSPECIFIED. ) 
 CURVE ( )  GEOMETRIC_REPRESENTATION_ITEM ( )  RATIONAL_B_SPLINE_CURVE ( ( 0.9330127018922194093, 0.9330127018922194093, 1.000000000000000000, 0.8660254037844387076, 1.000000000000000000, 0.8660254037844387076, 1.000000000000000000, 0.9330127018922189652, 0.9330127018922194093 ) ) 
 REPRESENTATION_ITEM ( '' )  );
#8386=B_SPLINE_CURVE_WITH_KNOTS ( 'NONE', 1,
 ( #5123, #881 ),
 .UNSPECIFIED., .F., .F.,
 ( 2, 2 ),
 ( 0.000000000000000000, 1.000000000000000000 ),
 .UNSPECIFIED. ) ;
#8388=CARTESIAN_POINT ( 'NONE',  ( -25.98076211353311393, 55.53749999808803750, -2.690598923241634743 ) ) ;
#8390=ORIENTED_EDGE ( 'NONE', *, *, #4046, .T. ) ;
#8396=CARTESIAN_POINT ( 'NONE',  ( -25.98076211353311393, 49.49999999999986500, -3.000000000000131894 ) ) ;
#8405=AXIS2_PLACEMENT_3D ( 'NONE', #10713, #4733, #8110 ) ;
#8408=DIRECTION ( 'NONE',  ( 0.000000000000000000, 1.000000000000000000, 0.000000000000000000 ) ) ;
#8412=CARTESIAN_POINT ( 'NONE',  ( -26.79131905728310059, 50.18541666571061199, -3.596074190997381237 ) ) ;
#8417=CARTESIAN_POINT ( 'NONE',  ( -25.98076211353311393, 50.72499999999985931, -3.000000000000132783 ) ) ;
#8419=CARTESIAN_POINT ( 'NONE',  ( -27.98076211353308551, 53.20416666475470180, -6.154700538379338504 ) ) ;
#8421=CARTESIAN_POINT ( 'NONE',  ( -26.79131905728310059, 52.46041666571061768, -3.596074190997381237 ) ) ;
#8426=CARTESIAN_POINT ( 'NONE',  ( -27.98076211353308551, 51.19166666666652787, -6.154700538379338504 ) ) ;
#8431=ORIENTED_EDGE ( 'NONE', *, *, #6409, .T. ) ;
#8438=( BOUNDED_CURVE ( )  B_SPLINE_CURVE ( 2, ( #6685, #4307, #7697, #3475, #7464, #10084, #8297, #682, #2473 ),
 .UNSPECIFIED., .F., .F. ) 
 B_SPLINE_CURVE_WITH_KNOTS ( ( 3, 2, 2, 2, 3 ),
 ( 0.3611111111111111049, 0.3703703703703703498, 0.3888888888888888951, 0.4074074074074073848, 0.4166666666666666297 ),
 .UNSPECIFIED. ) 
 CURVE ( )  GEOMETRIC_REPRESENTATION_ITEM ( )  RATIONAL_B_SPLINE_CURVE ( ( 0.9330127018922194093, 0.9330127018922194093, 1.000000000000000000, 0.8660254037844387076, 1.000000000000000000, 0.8660254037844387076, 1.000000000000000000, 0.9330127018922196314, 0.9330127018922194093 ) ) 
 REPRESENTATION_ITEM ( '' )  );
#8441=AXIS2_PLACEMENT_3D ( 'NONE', #8916, #7346, #3860 ) ;
#8443=CARTESIAN_POINT ( 'NONE',  ( -26.79131905728310059, 50.36041666571060915, -3.596074190997381237 ) ) ;
#8444=EDGE_CURVE ( 'NONE', #6740, #10232, #10550, .T. ) ;
#8448=CARTESIAN_POINT ( 'NONE',  ( -25.17020516978313083, 50.01041666571061484, -6.403925809002825709 ) ) ;
#8452=CARTESIAN_POINT ( 'NONE',  ( -25.47444609516507441, 58.87210758029105762, -3.061288170098404926 ) ) ;
#8460=CARTESIAN_POINT ( 'NONE',  ( -27.60187600103308014, 52.22708333237728340, -4.064049460664955760 ) ) ;
#8469=CARTESIAN_POINT ( 'NONE',  ( -25.98076211353311393, 49.49999999999986500, -5.000000000000103029 ) ) ;
#8475=CARTESIAN_POINT ( 'NONE',  ( -25.98076211353311393, 52.69374999904394485, -6.871901078670400231 ) ) ;
#8483=CARTESIAN_POINT ( 'NONE',  ( -26.79131905728310059, 54.56041666571061199, -3.596074190997381237 ) ) ;
#8484=CARTESIAN_POINT ( 'NONE',  ( -27.60187600103308014, 55.69181177618368395, -4.629976867109323990 ) ) ;
#8488=CARTESIAN_POINT ( 'NONE',  ( -24.98076211353312814, 52.41666666666652930, -6.732050807568954909 ) ) ;
#8489=VERTEX_POINT ( 'NONE', #1218 ) ;
#8492=ORIENTED_EDGE ( 'NONE', *, *, #3844, .F. ) ;
#8495=ORIENTED_EDGE ( 'NONE', *, *, #7977, .T. ) ;
#8500=CARTESIAN_POINT ( 'NONE',  ( -27.98076211353308551, 51.86249999808803324, -5.000000000000103029 ) ) ;
#8505=CARTESIAN_POINT ( 'NONE',  ( -27.98076211353308551, 55.30416666475468901, -6.154700538379338504 ) ) ;
#8508=CARTESIAN_POINT ( 'NONE',  ( -25.98076211353311393, 50.63749999808803892, -3.000000000000132339 ) ) ;
#8510=ORIENTED_EDGE ( 'NONE', *, *, #4990, .F. ) ;
#8514=EDGE_CURVE ( 'NONE', #9774, #4274, #9176, .T. ) ;
#8517=ADVANCED_FACE ( 'NONE', ( #1952 ), #6382, .T. ) ;
#8520=CARTESIAN_POINT ( 'NONE',  ( -25.98076211353415843, 59.00000000000900968, -2.999999999996041389 ) ) ;
#8534=CARTESIAN_POINT ( 'NONE',  ( -25.98076211353311393, 53.04374999904395338, -3.128098921329806714 ) ) ;
#8541=CIRCLE ( 'NONE', #5657, 1.999999999999971356 ) ;
#8542=CARTESIAN_POINT ( 'NONE',  ( -25.17020516978313083, 54.91041666571061342, -6.403925809002825709 ) ) ;
#8546=CARTESIAN_POINT ( 'NONE',  ( -23.98076211353314235, 50.95833333333318649, -6.154700538379337615 ) ) ;
#8557=PLANE ( 'NONE',  #7317 ) ;
#8558=CARTESIAN_POINT ( 'NONE',  ( -27.60187600103308014, 50.18541666571061199, -5.935950539335252074 ) ) ;
#8559=CARTESIAN_POINT ( 'NONE',  ( -24.98076211353312814, 53.81666666666652787, -6.732050807568954909 ) ) ;
#8562=VERTEX_POINT ( 'NONE', #7425 ) ;
#8570=CARTESIAN_POINT ( 'NONE',  ( -25.98076211353311393, 49.89374999904395480, -6.871901078670400231 ) ) ;
#8571=PRODUCT_DEFINITION ( 'UNKNOWN', '', #2981, #4116 ) ;
#8580=CARTESIAN_POINT ( 'NONE',  ( -26.51666049839534622, 52.50626073911683278, -7.000000000000073719 ) ) ;
#8581=EDGE_CURVE ( 'NONE', #3184, #3474, #10815, .T. ) ;
#8583=CARTESIAN_POINT ( 'NONE',  ( -25.98076211353311393, 54.09374999904395054, -6.871901078670400231 ) ) ;
#8588=ORIENTED_EDGE ( 'NONE', *, *, #8238, .T. ) ;
#8591=CARTESIAN_POINT ( 'NONE',  ( -26.51666049839534622, 53.11876073720499392, -7.000000000000073719 ) ) ;
#8592=CARTESIAN_POINT ( 'NONE',  ( -25.17020516978313083, 53.97708333237728340, -3.596074190997380349 ) ) ;
#8594=CARTESIAN_POINT ( 'NONE',  ( -25.17020516978313083, 55.43541666571061910, -6.403925809002825709 ) ) ;
#8603=EDGE_CURVE ( 'NONE', #1390, #1944, #260, .T. ) ;
#8617=CARTESIAN_POINT ( 'NONE',  ( -25.17020516978313083, 51.17708333237727913, -3.596074190997380349 ) ) ;
#8620=ORIENTED_EDGE ( 'NONE', *, *, #4458, .F. ) ;
#8630=CARTESIAN_POINT ( 'NONE',  ( -24.35964822603314417, 51.81874999904395196, -5.000000000000103029 ) ) ;
#8639=EDGE_CURVE ( 'NONE', #1738, #7809, #4133, .T. ) ;
#8642=CARTESIAN_POINT ( 'NONE',  ( -25.98076211353311393, 55.14374999904394059, -3.128098921329806714 ) ) ;
#8644=CARTESIAN_POINT ( 'NONE',  ( -24.98076211353193798, 57.99999999999910472, -3.267949192431741423 ) ) ;
#8654=CARTESIAN_POINT ( 'NONE',  ( -26.79131905728310059, 55.02708333237728056, -6.403925809002825709 ) ) ;
#8655=CARTESIAN_POINT ( 'NONE',  ( -25.44486372867087454, 54.95626073911682852, -3.000000000000134559 ) ) ;
#8671=EDGE_CURVE ( 'NONE', #2510, #3184, #4943, .T. ) ;
#8675=CARTESIAN_POINT ( 'NONE',  ( -26.79131905728310059, 51.52708333237728056, -6.403925809002825709 ) ) ;
#8683=VERTEX_POINT ( 'NONE', #1310 ) ;
#8685=DIRECTION ( 'NONE',  ( 0.000000000000000000, 0.000000000000000000, 1.000000000000000000 ) ) ;
#8687=CARTESIAN_POINT ( 'NONE',  ( -26.79131905728310059, 51.35208333237728340, -6.403925809002825709 ) ) ;
#8700=DIRECTION ( 'NONE',  ( 0.000000000000000000, 1.000000000000000000, 0.000000000000000000 ) ) ;
#8707=CARTESIAN_POINT ( 'NONE',  ( -24.98076211353312814, 53.72916666475470038, -6.732050807568954909 ) ) ;
#8709=CARTESIAN_POINT ( 'NONE',  ( -23.98076211353314235, 55.04166666666652930, -3.845299461620867554 ) ) ;
#8713=EDGE_CURVE ( 'NONE', #6644, #9280, #3432, .T. ) ;
#8714=DIRECTION ( 'NONE',  ( 0.000000000000000000, 1.000000000000000000, 0.000000000000000000 ) ) ;
#8724=CARTESIAN_POINT ( 'NONE',  ( -27.60187600103308014, 53.68541666571061199, -5.935950539335252074 ) ) ;
#8729=ORIENTED_EDGE ( 'NONE', *, *, #7443, .T. ) ;
#8735=CARTESIAN_POINT ( 'NONE',  ( -25.98076211353311393, 55.14374999904394059, -3.128098921329806714 ) ) ;
#8738=DIRECTION ( 'NONE',  ( 0.000000000000000000, 1.000000000000000000, 0.000000000000000000 ) ) ;
#8745=( BOUNDED_CURVE ( )  B_SPLINE_CURVE ( 2, ( #2936, #3707, #6312, #3653, #5324, #10488, #2100, #8877, #1261 ),
 .UNSPECIFIED., .F., .F. ) 
 B_SPLINE_CURVE_WITH_KNOTS ( ( 3, 2, 2, 2, 3 ),
 ( 0.5277777777777777901, 0.5370370370370370905, 0.5555555555555555802, 0.5740740740740740700, 0.5833333333333333703 ),
 .UNSPECIFIED. ) 
 CURVE ( )  GEOMETRIC_REPRESENTATION_ITEM ( )  RATIONAL_B_SPLINE_CURVE ( ( 0.9330127018922194093, 0.9330127018922194093, 1.000000000000000000, 0.8660254037844387076, 1.000000000000000000, 0.8660254037844387076, 1.000000000000000000, 0.9330127018922189652, 0.9330127018922194093 ) ) 
 REPRESENTATION_ITEM ( '' )  );
#8747=CARTESIAN_POINT ( 'NONE',  ( -27.60187600103308370, 55.66874999904394627, -5.000000000000103029 ) ) ;
#8759=CARTESIAN_POINT ( 'NONE',  ( -24.35964822603314772, 52.05208333237727913, -5.935950539335252074 ) ) ;
#8761=CARTESIAN_POINT ( 'NONE',  ( -24.98076211353312814, 54.51666666666653072, -6.732050807568954909 ) ) ;
#8764=CARTESIAN_POINT ( 'NONE',  ( -26.98076211353309972, 54.63333333333319786, -6.732050807568954909 ) ) ;
#8766=FACE_OUTER_BOUND ( 'NONE', #9915, .T. ) ;
#8775=CARTESIAN_POINT ( 'NONE',  ( -27.60187600103308014, 51.70208333237727771, -4.064049460664955760 ) ) ;
#8783=SHAPE_REPRESENTATION_RELATIONSHIP ( 'NONE' , 'NONE' ,  #5283, #3752 ) ;
#8785=EDGE_CURVE ( 'NONE', #8489, #276, #1148, .T. ) ;
#8790=CARTESIAN_POINT ( 'NONE',  ( -24.35964822603314772, 53.97708333237728340, -5.935950539335252074 ) ) ;
#8801=CARTESIAN_POINT ( 'NONE',  ( -25.98076211353311393, 50.02499999999987068, -3.000000000000132783 ) ) ;
#8805=CARTESIAN_POINT ( 'NONE',  ( -25.98076211353311749, 56.99999999999884182, -7.000000000000094147 ) ) ;
#8812=ORIENTED_EDGE ( 'NONE', *, *, #2748, .F. ) ;
#8816=CARTESIAN_POINT ( 'NONE',  ( -26.51666049839534978, 53.40623925897106972, -3.000000000000133227 ) ) ;
#8818=( BOUNDED_CURVE ( )  B_SPLINE_CURVE ( 2, ( #4433, #8580, #964, #4371, #7815, #7756, #137, #3537, #5257 ),
 .UNSPECIFIED., .F., .F. ) 
 B_SPLINE_CURVE_WITH_KNOTS ( ( 3, 2, 2, 2, 3 ),
 ( 0.4722222222222222099, 0.4814814814814814548, 0.5000000000000000000, 0.5185185185185184897, 0.5277777777777777901 ),
 .UNSPECIFIED. ) 
 CURVE ( )  GEOMETRIC_REPRESENTATION_ITEM ( )  RATIONAL_B_SPLINE_CURVE ( ( 0.9330127018922194093, 0.9330127018922194093, 1.000000000000000000, 0.8660254037844387076, 1.000000000000000000, 0.8660254037844387076, 1.000000000000000000, 0.9330127018922194093, 0.9330127018922194093 ) ) 
 REPRESENTATION_ITEM ( '' )  );
#8819=CARTESIAN_POINT ( 'NONE',  ( -26.24705249213157288, 57.02715675374773951, -6.986049842788033537 ) ) ;
#8822=CARTESIAN_POINT ( 'NONE',  ( -25.17020516978313083, 52.57708333237728482, -3.596074190997380349 ) ) ;
#8824=CARTESIAN_POINT ( 'NONE',  ( -23.98076211353314235, 55.09999999999986642, -5.000000000000103029 ) ) ;
#8825=ORIENTED_EDGE ( 'NONE', *, *, #10223, .F. ) ;
#8830=CYLINDRICAL_SURFACE ( 'NONE', #10903, 4.000000000000599520 ) ;
#8838=CARTESIAN_POINT ( 'NONE',  ( -25.98076211353311393, 54.61874999904394912, -3.128098921329806714 ) ) ;
#8846=COLOUR_RGB ( '', 0.66274510, 0.83137255, 0.94901961) ;
#8848=SURFACE_STYLE_USAGE ( .BOTH. , #7072 ) ;
#8851=CARTESIAN_POINT ( 'NONE',  ( -26.98076211353309972, 49.73333333333319928, -6.732050807568954909 ) ) ;
#8854=CARTESIAN_POINT ( 'NONE',  ( -25.98076211353311393, 50.28749999808804461, -7.000000000000073719 ) ) ;
#8862=DIRECTION ( 'NONE',  ( 0.000000000000000000, 1.000000000000000000, 0.000000000000000000 ) ) ;
#8863=CARTESIAN_POINT ( 'NONE',  ( -25.44486372867087454, 50.05626073911682994, -3.000000000000132339 ) ) ;
#8872=VERTEX_POINT ( 'NONE', #1422 ) ;
#8873=EDGE_CURVE ( 'NONE', #4861, #9687, #6413, .T. ) ;
#8877=CARTESIAN_POINT ( 'NONE',  ( -25.44486372867087809, 53.14373926088290290, -7.000000000000075495 ) ) ;
#8879=CARTESIAN_POINT ( 'NONE',  ( -26.79131905728310059, 52.22708333237727629, -6.403925809002825709 ) ) ;
#8883=CARTESIAN_POINT ( 'NONE',  ( -24.98076211353313170, 50.69583333142136183, -3.267949192431250705 ) ) ;
#8890=CARTESIAN_POINT ( 'NONE',  ( -27.60187600103308014, 52.28541666571061342, -5.935950539335252074 ) ) ;
#8909=CARTESIAN_POINT ( 'NONE',  ( -26.24619511045171194, 58.97315198882180454, -3.013802259003559580 ) ) ;
#8912=CARTESIAN_POINT ( 'NONE',  ( -25.00808978981783781, 57.73360806846572757, -6.748470692696331596 ) ) ;
#8916=CARTESIAN_POINT ( 'NONE',  ( -25.98076211353311393, 49.49999999999986500, -5.000000000000103029 ) ) ;
#8924=CARTESIAN_POINT ( 'NONE',  ( -25.98076211353311393, 51.42499999999986926, -3.000000000000132339 ) ) ;
#8925=CARTESIAN_POINT ( 'NONE',  ( -25.17020516978313083, 53.27708333237728056, -3.596074190997380349 ) ) ;
#8933=DIRECTION ( 'NONE',  ( 0.000000000000000000, 1.000000000000000000, 0.000000000000000000 ) ) ;
#8935=CARTESIAN_POINT ( 'NONE',  ( -24.35964822603314417, 51.11874999904394912, -5.000000000000103029 ) ) ;
#8942=CYLINDRICAL_SURFACE ( 'NONE', #8405, 1.999999999999971356 ) ;
#8945=ORIENTED_EDGE ( 'NONE', *, *, #409, .T. ) ;
#8947=FILL_AREA_STYLE ('',( #4629 ) ) ;
#8952=CARTESIAN_POINT ( 'NONE',  ( -25.98076211353311393, 53.08749999808803466, -7.309401076758571314 ) ) ;
#8957=CLOSED_SHELL ( 'NONE', ( #7297, #3382, #7477, #4792, #4886, #8517, #6214, #4254, #7358, #5877, #8071, #8178, #3070, #2964, #4852, #3664, #7350, #6895, #4315, #7226, #4548, #7997, #7989, #7598, #2527, #6380, #6868, #902, #2613, #3025, #10853, #5403, #9956 ) ) ;
#8965=CIRCLE ( 'NONE', #6674, 3.500000000000591971 ) ;
#8975=VECTOR ( 'NONE', #1026, 1000.000000000000000 ) ;
#8981=CARTESIAN_POINT ( 'NONE',  ( -25.98076211353311393, 52.86874999904393491, -6.871901078670400231 ) ) ;
#8991=CARTESIAN_POINT ( 'NONE',  ( -24.35964822603314772, 51.93541666571061199, -4.064049460664953983 ) ) ;
#8993=CARTESIAN_POINT ( 'NONE',  ( -26.79131905728310059, 51.35208333237728340, -6.403925809002825709 ) ) ;
#8997=CARTESIAN_POINT ( 'NONE',  ( -25.17020516978313083, 55.61041666571061626, -6.403925809002825709 ) ) ;
#9004=EDGE_LOOP ( 'NONE', ( #1780, #8510, #4789, #8620 ) ) ;
#9008=( NAMED_UNIT ( * ) PLANE_ANGLE_UNIT ( ) SI_UNIT ( $, .RADIAN. ) );
#9011=CARTESIAN_POINT ( 'NONE',  ( -26.98076211353309972, 53.14583333142136468, -6.732050807568954909 ) ) ;
#9012=CIRCLE ( 'NONE', #315, 4.000000000000600409 ) ;
#9014=CARTESIAN_POINT ( 'NONE',  ( -25.98076211353311393, 53.78749999808803040, -7.000000000000072831 ) ) ;
#9017=VERTEX_POINT ( 'NONE', #6291 ) ;
#9022=CARTESIAN_POINT ( 'NONE',  ( -27.98076211353308196, 56.08556087358027753, -4.543513051204862485 ) ) ;
#9027=CARTESIAN_POINT ( 'NONE',  ( -26.98076211353309972, 55.47916666475470038, -3.267949192431252037 ) ) ;
#9034=CARTESIAN_POINT ( 'NONE',  ( -25.98076211353311393, 55.31874999904394485, -3.128098921329806714 ) ) ;
#9039=DIRECTION ( 'NONE',  ( 0.000000000000000000, 0.000000000000000000, 1.000000000000000000 ) ) ;
#9040=CARTESIAN_POINT ( 'NONE',  ( -24.35964822603314417, 50.59374999904394343, -5.000000000000103029 ) ) ;
#9041=CARTESIAN_POINT ( 'NONE',  ( -27.60187600103308725, 55.02708333237728056, -4.064049460664955760 ) ) ;
#9043=CARTESIAN_POINT ( 'NONE',  ( -24.35964822603314772, 55.37708333237728198, -5.935950539335252074 ) ) ;
#9045=CARTESIAN_POINT ( 'NONE',  ( -27.60187600103308014, 55.78541666571062052, -5.935950539335252074 ) ) ;
#9048=EDGE_LOOP ( 'NONE', ( #8007, #8431, #8825, #5276 ) ) ;
#9056=CARTESIAN_POINT ( 'NONE',  ( -24.98076211353312814, 53.72916666475470038, -6.732050807568954909 ) ) ;
#9063=EDGE_CURVE ( 'NONE', #9687, #10877, #7616, .T. ) ;
#9066=CARTESIAN_POINT ( 'NONE',  ( -24.35964822603314417, 49.71874999904395054, -5.000000000000103029 ) ) ;
#9067=CARTESIAN_POINT ( 'NONE',  ( -25.98076211353311393, 49.49999999999986500, -5.000000000000103029 ) ) ;
#9078=LINE ( 'NONE', #3366, #10137 ) ;
#9079=CARTESIAN_POINT ( 'NONE',  ( -27.60187600103308014, 55.78541666571062052, -5.935950539335252074 ) ) ;
#9083=VERTEX_POINT ( 'NONE', #2137 ) ;
#9087=CARTESIAN_POINT ( 'NONE',  ( -27.60187600103308370, 50.94374999904394485, -5.000000000000103029 ) ) ;
#9088=CARTESIAN_POINT ( 'NONE',  ( -25.17020516978313083, 54.03541666571061342, -6.403925809002825709 ) ) ;
#9090=CARTESIAN_POINT ( 'NONE',  ( -24.98076211353312814, 50.31666666666652787, -6.732050807568954909 ) ) ;
#9091=ORIENTED_EDGE ( 'NONE', *, *, #8603, .F. ) ;
#9092=CARTESIAN_POINT ( 'NONE',  ( -24.35964822603314417, 55.49374999904394912, -5.000000000000103029 ) ) ;
#9094=ORIENTED_EDGE ( 'NONE', *, *, #10382, .T. ) ;
#9096=ORIENTED_EDGE ( 'NONE', *, *, #9594, .F. ) ;
#9097=DIRECTION ( 'NONE',  ( 2.775557561562891351E-17, 1.000000000000000000, -8.326672684688671588E-17 ) ) ;
#9105=CARTESIAN_POINT ( 'NONE',  ( -27.98076211353308551, 51.16249999808803750, -5.000000000000103029 ) ) ;
#9117=FACE_OUTER_BOUND ( 'NONE', #3936, .T. ) ;
#9127=DIRECTION ( 'NONE',  ( 0.000000000000000000, 0.000000000000000000, 1.000000000000000000 ) ) ;
#9134=CARTESIAN_POINT ( 'NONE',  ( -27.60187600103308014, 50.71041666571061768, -5.935950539335252074 ) ) ;
#9135=CARTESIAN_POINT ( 'NONE',  ( -25.98076211353311393, 49.49999999999986500, -5.000000000000103029 ) ) ;
#9142=CARTESIAN_POINT ( 'NONE',  ( -25.98076211353310683, 51.11874999904394201, -3.128098921329806714 ) ) ;
#9143=CARTESIAN_POINT ( 'NONE',  ( -25.17020516978313083, 53.33541666571061768, -6.403925809002825709 ) ) ;
#9146=CARTESIAN_POINT ( 'NONE',  ( -26.98076211353309972, 52.53333333333319644, -6.732050807568954909 ) ) ;
#9147=ORIENTED_EDGE ( 'NONE', *, *, #3231, .F. ) ;
#9162=CARTESIAN_POINT ( 'NONE',  ( -27.98076211353308551, 53.20416666475470180, -6.154700538379338504 ) ) ;
#9163=CARTESIAN_POINT ( 'NONE',  ( -26.51666049839534622, 53.49373926088289721, -3.000000000000131006 ) ) ;
#9173=AXIS2_PLACEMENT_3D ( 'NONE', #5355, #8738, #1122 ) ;
#9176=B_SPLINE_CURVE_WITH_KNOTS ( 'NONE', 3,
 ( #3720, #4666, #7107, #3004 ),
 .UNSPECIFIED., .F., .F.,
 ( 4, 4 ),
 ( 0.000000000000000000, 1.000000000000000000 ),
 .UNSPECIFIED. ) ;
#9190=PLANE ( 'NONE',  #10316 ) ;
#9191=CARTESIAN_POINT ( 'NONE',  ( -26.79131905728310059, 54.56041666571061199, -3.596074190997381237 ) ) ;
#9196=B_SPLINE_CURVE_WITH_KNOTS ( 'NONE', 3,
 ( #9285, #9454, #1847, #4297, #6675, #5901, #6846, #5080, #2638, #10898 ),
 .UNSPECIFIED., .F., .F.,
 ( 4, 2, 2, 2, 4 ),
 ( 0.004768944099797328175, 0.005165600962498952294, 0.005562257825200575545, 0.005958914687902199664, 0.006355571550603823783 ),
 .UNSPECIFIED. ) ;
#9198=VECTOR ( 'NONE', #9961, 1000.000000000000000 ) ;
#9201=CARTESIAN_POINT ( 'NONE',  ( -26.79131905728310059, 51.76041666571061484, -3.596074190997381237 ) ) ;
#9202=CARTESIAN_POINT ( 'NONE',  ( -26.79131905728310059, 54.15208333237728056, -6.403925809002825709 ) ) ;
#9204=CARTESIAN_POINT ( 'NONE',  ( -27.98076211353308551, 53.29166666666653640, -6.154700538379338504 ) ) ;
#9206=CARTESIAN_POINT ( 'NONE',  ( -26.51666049839534622, 54.10623925897106545, -3.000000000000131006 ) ) ;
#9221=CARTESIAN_POINT ( 'NONE',  ( -25.98076211353311393, 50.06874999904394485, -6.871901078670400231 ) ) ;
#9233=CARTESIAN_POINT ( 'NONE',  ( -25.44486372867087454, 51.65623925897107682, -7.000000000000073719 ) ) ;
#9245=CARTESIAN_POINT ( 'NONE',  ( -25.17020516978313083, 54.91041666571061342, -6.403925809002825709 ) ) ;
#9252=CARTESIAN_POINT ( 'NONE',  ( -26.98076211353309972, 53.14583333142136468, -6.732050807568954909 ) ) ;
#9254=CARTESIAN_POINT ( 'NONE',  ( -27.60187600103308725, 55.20208333237727771, -4.064049460664955760 ) ) ;
#9255=CARTESIAN_POINT ( 'NONE',  ( -25.17020516978313083, 52.63541666571061484, -6.403925809002825709 ) ) ;
#9258=CARTESIAN_POINT ( 'NONE',  ( -27.98076211353308551, 53.40833333333319644, -3.845299461620869330 ) ) ;
#9261=EDGE_LOOP ( 'NONE', ( #10046, #10950, #1902, #6287, #10236, #957 ) ) ;
#9272=CARTESIAN_POINT ( 'NONE',  ( -24.35964822603314772, 49.95208333237727771, -5.935950539335252074 ) ) ;
#9276=CARTESIAN_POINT ( 'NONE',  ( -27.98076211353308551, 54.72083333142136041, -3.845299461620869330 ) ) ;
#9279=CARTESIAN_POINT ( 'NONE',  ( -26.98076211353309972, 50.57916666475469469, -3.267949192431252037 ) ) ;
#9280=VERTEX_POINT ( 'NONE', #1722 ) ;
#9285=CARTESIAN_POINT ( 'NONE',  ( -25.98076211353311393, 59.00000000000083134, -7.000000000000074607 ) ) ;
#9287=CARTESIAN_POINT ( 'NONE',  ( -27.60187600103308370, 51.46874999904395054, -5.000000000000103029 ) ) ;
#9292=ORIENTED_EDGE ( 'NONE', *, *, #553, .T. ) ;
#9298=DIRECTION ( 'NONE',  ( 2.775557561562891351E-17, 1.000000000000000000, -8.326672684688671588E-17 ) ) ;
#9299=CARTESIAN_POINT ( 'NONE',  ( -25.17020516978313083, 54.73541666571062336, -6.403925809002825709 ) ) ;
#9305=CARTESIAN_POINT ( 'NONE',  ( -27.98076211353308551, 50.49166666666652503, -6.154700538379338504 ) ) ;
#9306=EDGE_CURVE ( 'NONE', #10078, #6093, #8383, .T. ) ;
#9307=DIRECTION ( 'NONE',  ( 0.000000000000000000, 0.000000000000000000, 1.000000000000000000 ) ) ;
#9308=AXIS2_PLACEMENT_3D ( 'NONE', #5976, #7647, #3591 ) ;
#9309=CARTESIAN_POINT ( 'NONE',  ( -26.79131905728310059, 53.62708333237727487, -6.403925809002825709 ) ) ;
#9314=CARTESIAN_POINT ( 'NONE',  ( -27.98076211353308551, 53.99166666666653214, -6.154700538379338504 ) ) ;
#9335=EDGE_CURVE ( 'NONE', #2292, #8489, #6531, .T. ) ;
#9336=CARTESIAN_POINT ( 'NONE',  ( -26.98076211353309972, 54.07916666475470180, -3.267949192431252037 ) ) ;
#9348=CARTESIAN_POINT ( 'NONE',  ( -27.60187600103308370, 52.16874999904395338, -5.000000000000103029 ) ) ;
#9353=CARTESIAN_POINT ( 'NONE',  ( -26.98076211353408027, 58.06623402467567274, -6.732050807568390027 ) ) ;
#9364=CARTESIAN_POINT ( 'NONE',  ( -26.79131905728310059, 53.68541666571061910, -3.596074190997381237 ) ) ;
#9366=FACE_OUTER_BOUND ( 'NONE', #2078, .T. ) ;
#9372=CARTESIAN_POINT ( 'NONE',  ( -27.60187600103308370, 52.34374999904394343, -5.000000000000103029 ) ) ;
#9377=CARTESIAN_POINT ( 'NONE',  ( -27.98076211353308551, 50.54999999999986926, -5.000000000000103029 ) ) ;
#9383=ORIENTED_EDGE ( 'NONE', *, *, #754, .F. ) ;
#9385=DIRECTION ( 'NONE',  ( 8.659560562355001884E-17, -0.7071067811865420216, 0.7071067811865531239 ) ) ;
#9389=DIRECTION ( 'NONE',  ( 0.000000000000000000, 0.000000000000000000, 1.000000000000000000 ) ) ;
#9390=CARTESIAN_POINT ( 'NONE',  ( -25.98076211353311393, 50.76874999904394770, -6.871901078670400231 ) ) ;
#9393=LINE ( 'NONE', #6779, #2998 ) ;
#9402=CARTESIAN_POINT ( 'NONE',  ( -25.17020516978313083, 50.30208333237728624, -3.596074190997380349 ) ) ;
#9414=CARTESIAN_POINT ( 'NONE',  ( -25.98076211353311393, 52.34374999904395054, -3.128098921329806714 ) ) ;
#9419=ORIENTED_EDGE ( 'NONE', *, *, #9806, .F. ) ;
#9420=CARTESIAN_POINT ( 'NONE',  ( -27.98076211353308551, 54.02083333142136468, -3.845299461620869330 ) ) ;
#9421=B_SPLINE_CURVE_WITH_KNOTS ( 'NONE', 3,
 ( #1464, #6677, #6610, #2346, #7572, #10733, #3128, #6734, #10012, #10962 ),
 .UNSPECIFIED., .F., .F.,
 ( 4, 2, 2, 2, 4 ),
 ( 0.004769787300783674168, 0.005166447011858126687, 0.005563106722932580073, 0.005959766434007033459, 0.006356426145081485977 ),
 .UNSPECIFIED. ) ;
#9422=CARTESIAN_POINT ( 'NONE',  ( -26.51666049839535688, 50.40626073911683847, -7.000000000000074607 ) ) ;
#9424=CARTESIAN_POINT ( 'NONE',  ( -25.98076211353310683, 53.56874999904394485, -6.871901078670399343 ) ) ;
#9429=CARTESIAN_POINT ( 'NONE',  ( -27.78268512908117671, 55.49961679590671793, -4.132201955500060642 ) ) ;
#9442=CARTESIAN_POINT ( 'NONE',  ( -26.98076211353309972, 53.84583333142136752, -6.732050807568954909 ) ) ;
#9452=EDGE_CURVE ( 'NONE', #1598, #5575, #9601, .T. ) ;
#9454=CARTESIAN_POINT ( 'NONE',  ( -25.84843596800915932, 59.00000000000083844, -7.000000000000073719 ) ) ;
#9458=( BOUNDED_CURVE ( )  B_SPLINE_CURVE ( 2, ( #6931, #8655, #1034, #4445, #7825, #200, #6986, #10371, #2605 ),
 .UNSPECIFIED., .F., .F. ) 
 B_SPLINE_CURVE_WITH_KNOTS ( ( 3, 2, 2, 2, 3 ),
 ( 0.8611111111111111605, 0.8703703703703703498, 0.8888888888888888395, 0.9074074074074074403, 0.9166666666666667407 ),
 .UNSPECIFIED. ) 
 CURVE ( )  GEOMETRIC_REPRESENTATION_ITEM ( )  RATIONAL_B_SPLINE_CURVE ( ( 0.9330127018922194093, 0.9330127018922197424, 1.000000000000000000, 0.8660254037844387076, 1.000000000000000000, 0.8660254037844387076, 1.000000000000000000, 0.9330127018922189652, 0.9330127018922194093 ) ) 
 REPRESENTATION_ITEM ( '' )  );
#9466=CYLINDRICAL_SURFACE ( 'NONE', #3821, 1.999999999999971356 ) ;
#9468=CARTESIAN_POINT ( 'NONE',  ( -24.98076211353312814, 55.82916666475470180, -6.732050807568954909 ) ) ;
#9470=CARTESIAN_POINT ( 'NONE',  ( -25.98076211353311393, 53.39374999904394770, -6.871901078670400231 ) ) ;
#9472=CARTESIAN_POINT ( 'NONE',  ( -24.98076211353223641, 57.86679757347771158, -3.267949192431767180 ) ) ;
#9474=EDGE_CURVE ( 'NONE', #2370, #6817, #5410, .T. ) ;
#9480=CARTESIAN_POINT ( 'NONE',  ( -24.35964822603314417, 54.09374999904395054, -5.000000000000103029 ) ) ;
#9481=CARTESIAN_POINT ( 'NONE',  ( -27.60187600103308725, 55.61041666571062336, -5.935950539335252074 ) ) ;
#9485=ORIENTED_EDGE ( 'NONE', *, *, #9957, .F. ) ;
#9493=CARTESIAN_POINT ( 'NONE',  ( -25.44486372867087809, 54.54373926088290858, -7.000000000000075495 ) ) ;
#9496=EDGE_CURVE ( 'NONE', #8683, #10232, #9947, .T. ) ;
#9500=CARTESIAN_POINT ( 'NONE',  ( -24.35964822603314772, 51.93541666571061199, -4.064049460664953983 ) ) ;
#9501=AXIS2_PLACEMENT_3D ( 'NONE', #10858, #2308, #4024 ) ;
#9513=CARTESIAN_POINT ( 'NONE',  ( -25.98076211353311393, 51.29374999904394627, -6.871901078670400231 ) ) ;
#9522=CARTESIAN_POINT ( 'NONE',  ( -25.44486372867087454, 50.34373926088291284, -7.000000000000073719 ) ) ;
#9525=( BOUNDED_CURVE ( )  B_SPLINE_CURVE ( 2, ( #2219, #536, #5614, #8161, #9532, #9420, #5263, #9206, #6035 ),
 .UNSPECIFIED., .F., .T. ) 
 B_SPLINE_CURVE_WITH_KNOTS ( ( 3, 2, 2, 2, 3 ),
 ( 0.5833333333333333703, 0.5925925925925925597, 0.6111111111111111605, 0.6296296296296296502, 0.6388888888888889506 ),
 .UNSPECIFIED. ) 
 CURVE ( )  GEOMETRIC_REPRESENTATION_ITEM ( )  RATIONAL_B_SPLINE_CURVE ( ( 0.9330127018922194093, 0.9330127018922197424, 1.000000000000000000, 0.8660254037844387076, 1.000000000000000000, 0.8660254037844387076, 1.000000000000000000, 0.9330127018922189652, 0.9330127018922194093 ) ) 
 REPRESENTATION_ITEM ( '' )  );
#9527=CARTESIAN_POINT ( 'NONE',  ( -27.60187600103308014, 52.11041666571061626, -5.935950539335252074 ) ) ;
#9532=CARTESIAN_POINT ( 'NONE',  ( -27.98076211353308551, 53.96249999808803466, -5.000000000000103029 ) ) ;
#9538=CARTESIAN_POINT ( 'NONE',  ( -25.17020516978313083, 55.20208333237728482, -3.596074190997380349 ) ) ;
#9547=CARTESIAN_POINT ( 'NONE',  ( -24.98076211353312814, 50.92916666475470322, -6.732050807568954909 ) ) ;
#9553=CARTESIAN_POINT ( 'NONE',  ( -25.98076211353311393, 51.68749999808803608, -7.000000000000073719 ) ) ;
#9557=CARTESIAN_POINT ( 'NONE',  ( -26.79131905728310059, 52.22708333237727629, -6.403925809002825709 ) ) ;
#9559=ORIENTED_EDGE ( 'NONE', *, *, #5785, .T. ) ;
#9565=DIRECTION ( 'NONE',  ( 1.000000000000000000, 0.000000000000000000, 0.000000000000000000 ) ) ;
#9569=CARTESIAN_POINT ( 'NONE',  ( -25.98076211353311393, 54.79374999904395338, -6.871901078670400231 ) ) ;
#9573=ORIENTED_EDGE ( 'NONE', *, *, #1181, .F. ) ;
#9585=CARTESIAN_POINT ( 'NONE',  ( -26.98076211353309972, 53.37916666475469896, -3.267949192431252037 ) ) ;
#9586=EDGE_CURVE ( 'NONE', #2547, #9083, #10206, .T. ) ;
#9588=CARTESIAN_POINT ( 'NONE',  ( -24.35964822603314772, 54.15208333237728766, -5.935950539335252074 ) ) ;
#9591=EDGE_LOOP ( 'NONE', ( #54, #1723 ) ) ;
#9594=EDGE_CURVE ( 'NONE', #3608, #8338, #9458, .T. ) ;
#9599=CARTESIAN_POINT ( 'NONE',  ( -25.98076211353311393, 49.49999999999986500, -7.000000000000074607 ) ) ;
#9601=LINE ( 'NONE', #5554, #9849 ) ;
#9604=CARTESIAN_POINT ( 'NONE',  ( -25.98076211353311393, 52.86874999904393491, -6.871901078670400231 ) ) ;
#9620=CARTESIAN_POINT ( 'NONE',  ( -24.35964822603314417, 53.21874999904395764, -5.000000000000103029 ) ) ;
#9625=ORIENTED_EDGE ( 'NONE', *, *, #3404, .F. ) ;
#9631=CARTESIAN_POINT ( 'NONE',  ( -23.98076211353314235, 49.49999999999986500, -5.000000000000103029 ) ) ;
#9633=CARTESIAN_POINT ( 'NONE',  ( -26.98076211353309972, 52.44583333142136894, -6.732050807568954909 ) ) ;
#9641=( BOUNDED_CURVE ( )  B_SPLINE_CURVE ( 2, ( #6837, #5892, #3341, #4234, #5179, #4345, #8559, #6901, #2084 ),
 .UNSPECIFIED., .F., .F. ) 
 B_SPLINE_CURVE_WITH_KNOTS ( ( 3, 2, 2, 2, 3 ),
 ( 0.6388888888888889506, 0.6481481481481481399, 0.6666666666666666297, 0.6851851851851852304, 0.6944444444444445308 ),
 .UNSPECIFIED. ) 
 CURVE ( )  GEOMETRIC_REPRESENTATION_ITEM ( )  RATIONAL_B_SPLINE_CURVE ( ( 0.9330127018922194093, 0.9330127018922197424, 1.000000000000000000, 0.8660254037844387076, 1.000000000000000000, 0.8660254037844387076, 1.000000000000000000, 0.9330127018922189652, 0.9330127018922194093 ) ) 
 REPRESENTATION_ITEM ( '' )  );
#9647=CARTESIAN_POINT ( 'NONE',  ( -26.79131905728310059, 52.46041666571061768, -3.596074190997381237 ) ) ;
#9649=CARTESIAN_POINT ( 'NONE',  ( -27.98076211353308551, 54.80833333333318791, -3.845299461620869330 ) ) ;
#9650=ORIENTED_EDGE ( 'NONE', *, *, #6361, .F. ) ;
#9653=FACE_OUTER_BOUND ( 'NONE', #7994, .T. ) ;
#9658=CARTESIAN_POINT ( 'NONE',  ( -26.79131905728310059, 50.65208333237728766, -6.403925809002825709 ) ) ;
#9664=CARTESIAN_POINT ( 'NONE',  ( -26.79131905728310059, 54.56041666571061199, -3.596074190997381237 ) ) ;
#9669=ORIENTED_EDGE ( 'NONE', *, *, #1181, .T. ) ;
#9672=VECTOR ( 'NONE', #9385, 999.9999999999998863 ) ;
#9673=EDGE_CURVE ( 'NONE', #2508, #4738, #8745, .T. ) ;
#9678=CARTESIAN_POINT ( 'NONE',  ( -25.98076211353311393, 53.04374999904395338, -3.128098921329806714 ) ) ;
#9683=CARTESIAN_POINT ( 'NONE',  ( -25.98076211353311393, 54.57499999999986073, -7.000000000000072831 ) ) ;
#9687=VERTEX_POINT ( 'NONE', #9749 ) ;
#9688=FACE_OUTER_BOUND ( 'NONE', #6482, .T. ) ;
#9689=CARTESIAN_POINT ( 'NONE',  ( -23.98076211353314235, 50.19999999999986073, -5.000000000000103029 ) ) ;
#9691=CARTESIAN_POINT ( 'NONE',  ( -25.98076211353415843, 59.00000000000900968, -2.999999999996041389 ) ) ;
#9696=CARTESIAN_POINT ( 'NONE',  ( -25.98076211353310683, 54.92499999999986926, -3.000000000000132339 ) ) ;
#9706=CARTESIAN_POINT ( 'NONE',  ( -25.98076211353311393, 51.46874999904394343, -6.871901078670400231 ) ) ;
#9711=CARTESIAN_POINT ( 'NONE',  ( -27.98076211353308551, 54.74999999999985789, -5.000000000000103029 ) ) ;
#9712=DIRECTION ( 'NONE',  ( 0.000000000000000000, 0.000000000000000000, 1.000000000000000000 ) ) ;
#9721=CARTESIAN_POINT ( 'NONE',  ( -27.60187600103308014, 53.10208333237727629, -4.064049460664955760 ) ) ;
#9732=EDGE_CURVE ( 'NONE', #9017, #433, #4273, .T. ) ;
#9739=CARTESIAN_POINT ( 'NONE',  ( -25.98076211353311393, 53.87499999999986500, -7.000000000000072831 ) ) ;
#9749=CARTESIAN_POINT ( 'NONE',  ( -25.98076211353311393, 50.02499999999987068, -3.000000000000132783 ) ) ;
#9760=CARTESIAN_POINT ( 'NONE',  ( -23.98076211353314235, 53.55416666475470322, -3.845299461620867554 ) ) ;
#9762=DIRECTION ( 'NONE',  ( 0.000000000000000000, 1.000000000000000000, 0.000000000000000000 ) ) ;
#9763=CARTESIAN_POINT ( 'NONE',  ( -24.35964822603314772, 51.93541666571061199, -4.064049460664953983 ) ) ;
#9774=VERTEX_POINT ( 'NONE', #7468 ) ;
#9787=CARTESIAN_POINT ( 'NONE',  ( -27.98076211353308551, 52.50416666475469896, -6.154700538379338504 ) ) ;
#9796=CARTESIAN_POINT ( 'NONE',  ( -27.98076211353308551, 49.84999999999986642, -5.000000000000103029 ) ) ;
#9806=EDGE_CURVE ( 'NONE', #4566, #1598, #4726, .T. ) ;
#9814=CARTESIAN_POINT ( 'NONE',  ( -27.60187600103308370, 53.74374999904394201, -5.000000000000103029 ) ) ;
#9817=ORIENTED_EDGE ( 'NONE', *, *, #8873, .F. ) ;
#9818=( BOUNDED_CURVE ( )  B_SPLINE_CURVE ( 2, ( #3082, #6614, #2351, #782, #10850, #1468, #9027, #7349, #3241 ),
 .UNSPECIFIED., .F., .F. ) 
 B_SPLINE_CURVE_WITH_KNOTS ( ( 3, 2, 2, 2, 3 ),
 ( 0.8055555555555555802, 0.8148148148148147696, 0.8333333333333333703, 0.8518518518518518601, 0.8611111111111111605 ),
 .UNSPECIFIED. ) 
 CURVE ( )  GEOMETRIC_REPRESENTATION_ITEM ( )  RATIONAL_B_SPLINE_CURVE ( ( 0.9330127018922194093, 0.9330127018922197424, 1.000000000000000000, 0.8660254037844387076, 1.000000000000000000, 0.8660254037844387076, 1.000000000000000000, 0.9330127018922189652, 0.9330127018922194093 ) ) 
 REPRESENTATION_ITEM ( '' )  );
#9819=CARTESIAN_POINT ( 'NONE',  ( -24.98076211353312814, 54.42916666475469611, -6.732050807568954909 ) ) ;
#9825=CARTESIAN_POINT ( 'NONE',  ( -24.35964822603314417, 51.29374999904394627, -5.000000000000103029 ) ) ;
#9826=CARTESIAN_POINT ( 'NONE',  ( -27.60187600103308725, 50.01041666571062194, -5.935950539335252074 ) ) ;
#9828=EDGE_LOOP ( 'NONE', ( #9903, #6906, #5718, #10375 ) ) ;
#9834=EDGE_LOOP ( 'NONE', ( #5576, #2570, #3372, #6225, #9884, #6645, #9573, #9887, #2225, #10889 ) ) ;
#9836=( NAMED_UNIT ( * ) SI_UNIT ( $, .STERADIAN. ) SOLID_ANGLE_UNIT ( ) );
#9842=CARTESIAN_POINT ( 'NONE',  ( -26.98076211353309972, 51.27916666475469754, -3.267949192431252037 ) ) ;
#9849=VECTOR ( 'NONE', #4562, 999.9999999999998863 ) ;
#9852=CARTESIAN_POINT ( 'NONE',  ( -26.51666049839534978, 49.70626073911682141, -7.000000000000073719 ) ) ;
#9854=CARTESIAN_POINT ( 'NONE',  ( -25.18289562231869283, 57.38366758799607936, -6.836521581664483094 ) ) ;
#9869=CARTESIAN_POINT ( 'NONE',  ( -24.35964822603314772, 51.06041666571061199, -4.064049460664953983 ) ) ;
#9871=CARTESIAN_POINT ( 'NONE',  ( -27.78268512908116961, 55.49961679590672503, -4.132201955500060642 ) ) ;
#9873=VERTEX_POINT ( 'NONE', #4865 ) ;
#9874=CARTESIAN_POINT ( 'NONE',  ( -25.44486372867087809, 54.45623925897106687, -7.000000000000075495 ) ) ;
#9879=CARTESIAN_POINT ( 'NONE',  ( -27.60187600103308725, 53.51041666571062194, -5.935950539335252074 ) ) ;
#9882=( BOUNDED_CURVE ( )  B_SPLINE_CURVE ( 1, ( #239, #3638 ),
 .UNSPECIFIED., .F., .T. ) 
 B_SPLINE_CURVE_WITH_KNOTS ( ( 2, 2 ),
 ( 0.000000000000000000, 1.000000000000000000 ),
 .UNSPECIFIED. ) 
 CURVE ( )  GEOMETRIC_REPRESENTATION_ITEM ( )  RATIONAL_B_SPLINE_CURVE ( ( 0.9343185842653825013, 0.9343185842653825013 ) ) 
 REPRESENTATION_ITEM ( '' )  );
#9883=CARTESIAN_POINT ( 'NONE',  ( -26.79131905728310059, 54.85208333237729050, -6.403925809002825709 ) ) ;
#9884=ORIENTED_EDGE ( 'NONE', *, *, #9586, .T. ) ;
#9886=ORIENTED_EDGE ( 'NONE', *, *, #9732, .T. ) ;
#9887=ORIENTED_EDGE ( 'NONE', *, *, #6540, .F. ) ;
#9889=ORIENTED_EDGE ( 'NONE', *, *, #10142, .F. ) ;
#9898=CARTESIAN_POINT ( 'NONE',  ( -23.98076211353314235, 53.55416666475470322, -3.845299461620867554 ) ) ;
#9902=CARTESIAN_POINT ( 'NONE',  ( -26.98076211353309972, 51.04583333142137036, -6.732050807568954909 ) ) ;
#9903=ORIENTED_EDGE ( 'NONE', *, *, #3404, .T. ) ;
#9915=EDGE_LOOP ( 'NONE', ( #6965, #3892, #3143, #5438 ) ) ;
#9916=CYLINDRICAL_SURFACE ( 'NONE', #7947, 1.999999999999971356 ) ;
#9923=CARTESIAN_POINT ( 'NONE',  ( -24.35964822603314417, 54.79374999904394627, -5.000000000000103029 ) ) ;
#9926=ORIENTED_EDGE ( 'NONE', *, *, #5161, .F. ) ;
#9928=DIRECTION ( 'NONE',  ( 0.000000000000000000, 0.000000000000000000, 1.000000000000000000 ) ) ;
#9931=( BOUNDED_SURFACE ( )  B_SPLINE_SURFACE ( 1, 2, ( 
 ( #7631, #6910, #6960, #8570, #10348, #844, #2691, #5140, #2641, #6017, #9402, #3625, #6066, #952, #4356, #3575, #123, #2744, #3467, #3524, #7747, #1849, #10297, #5243, #10405, #6118, #5302, #9513, #8687, #1062, #9287, #7854, #229, #1680, #5082, #5960, #8630, #7015, #5904, #1008, #179, #4420, #9348, #8460, #62, #6, #3407, #6849, #7805, #6788, #10183, #2577, #897, #4299, #7689, #10242, #5189, #9678, #4044, #6181, #9620, #7076, #1967, #1235, #2016, #5405, #3103, #2911, #6281, #1119, #5351, #6481, #4521, #8790, #2273, #4632, #7962, #2803, #1484, #1435, #7319, #339, #7376, #10762, #6229, #7428, #3682, #9569, #9883, #2073, #646, #10707, #1174, #8735, #10465, #5664, #7909, #9043, #4831, #4576, #8206, #3735, #287, #7122, #10517 ),
 ( #2859, #8016, #5460, #9934, #8851, #8262, #388, #3791, #586, #3982, #3154, #6537, #2319, #5711, #9090, #4882, #3203, #5762, #9377, #1773, #925, #10209, #4147, #6759, #7660, #8546, #4096, #2489, #4327, #8426, #870, #3438, #10989, #10818, #8316, #5049, #6582, #7541, #5874, #4271, #5822, #5164, #4214, #10929, #3260, #9985, #1543, #2369, #747, #6641, #8488, #697, #9146, #4995, #3321, #808, #4946, #7483, #10871, #10045, #2432, #2608, #6707, #10157, #35, #9204, #1597, #9258, #8368, #7604, #6813, #5986, #3379, #10102, #1652, #2544, #5926, #9314, #1711, #5110, #2719, #2043, #1089, #4447, #154, #3711, #8761, #7101, #5377, #93, #1144, #9649, #3493, #6877, #7776, #8709, #8824, #10494, #4497, #1991, #256, #3550, #4553, #1883, #9429 ) ),
 .UNSPECIFIED., .F., .F., .T. ) 
 B_SPLINE_SURFACE_WITH_KNOTS ( ( 2, 2 ),
 ( 3, 2, 2, 2, 2, 2, 2, 2, 2, 2, 2, 2, 2, 2, 2, 2, 2, 2, 2, 2, 2, 2, 2, 2, 2, 2, 2, 2, 2, 2, 2, 2, 2, 2, 2, 2, 2, 2, 2, 2, 2, 2, 2, 2, 2, 2, 2, 2, 2, 2, 2, 2, 3 ),
 ( 0.000000000000000000, 1.000000000000000000 ),
 ( 0.000000000000000000, 0.01851851851851851749, 0.03703703703703703498, 0.05555555555555555247, 0.07407407407407406996, 0.09259259259259258745, 0.1111111111111111049, 0.1296296296296296224, 0.1481481481481481399, 0.1666666666666666574, 0.1851851851851851749, 0.2037037037037036924, 0.2222222222222222099, 0.2407407407407407274, 0.2592592592592592449, 0.2777777777777777901, 0.2962962962962962798, 0.3148148148148148251, 0.3333333333333333148, 0.3518518518518518601, 0.3703703703703703498, 0.3888888888888888951, 0.4074074074074073848, 0.4259259259259259300, 0.4444444444444444198, 0.4629629629629629650, 0.4814814814814814548, 0.5000000000000000000, 0.5185185185185184897, 0.5370370370370370905, 0.5555555555555555802, 0.5740740740740740700, 0.5925925925925925597, 0.6111111111111111605, 0.6296296296296296502, 0.6481481481481481399, 0.6666666666666666297, 0.6851851851851852304, 0.7037037037037037202, 0.7222222222222222099, 0.7407407407407406996, 0.7592592592592593004, 0.7777777777777777901, 0.7962962962962962798, 0.8148148148148147696, 0.8333333333333333703, 0.8518518518518518601, 0.8703703703703703498, 0.8888888888888888395, 0.9074074074074074403, 0.9259259259259259300, 0.9444444444444444198, 0.9524110019352027834 ),
 .UNSPECIFIED. ) 
 GEOMETRIC_REPRESENTATION_ITEM ( )  RATIONAL_B_SPLINE_SURFACE ( (
 ( 1.000000000000000000, 0.8660254037844387076, 1.000000000000000000, 0.8660254037844387076, 1.000000000000000000, 0.8660254037844387076, 1.000000000000000000, 0.8660254037844387076, 1.000000000000000000, 0.8660254037844387076, 1.000000000000000000, 0.8660254037844387076, 1.000000000000000000, 0.8660254037844387076, 1.000000000000000000, 0.8660254037844387076, 1.000000000000000000, 0.8660254037844387076, 1.000000000000000000, 0.8660254037844387076, 1.000000000000000000, 0.8660254037844387076, 1.000000000000000000, 0.8660254037844387076, 1.000000000000000000, 0.8660254037844387076, 1.000000000000000000, 0.8660254037844387076, 1.000000000000000000, 0.8660254037844387076, 1.000000000000000000, 0.8660254037844387076, 1.000000000000000000, 0.8660254037844387076, 1.000000000000000000, 0.8660254037844387076, 1.000000000000000000, 0.8660254037844387076, 1.000000000000000000, 0.8660254037844387076, 1.000000000000000000, 0.8660254037844387076, 1.000000000000000000, 0.8660254037844387076, 1.000000000000000000, 0.8660254037844387076, 1.000000000000000000, 0.8660254037844387076, 1.000000000000000000, 0.8660254037844387076, 1.000000000000000000, 0.8660254037844387076, 1.000000000000000000, 0.8660254037844387076, 1.000000000000000000, 0.8660254037844387076, 1.000000000000000000, 0.8660254037844387076, 1.000000000000000000, 0.8660254037844387076, 1.000000000000000000, 0.8660254037844387076, 1.000000000000000000, 0.8660254037844387076, 1.000000000000000000, 0.8660254037844387076, 1.000000000000000000, 0.8660254037844387076, 1.000000000000000000, 0.8660254037844387076, 1.000000000000000000, 0.8660254037844387076, 1.000000000000000000, 0.8660254037844387076, 1.000000000000000000, 0.8660254037844387076, 1.000000000000000000, 0.8660254037844387076, 1.000000000000000000, 0.8660254037844387076, 1.000000000000000000, 0.8660254037844387076, 1.000000000000000000, 0.8660254037844387076, 1.000000000000000000, 0.8660254037844387076, 1.000000000000000000, 0.8660254037844387076, 1.000000000000000000, 0.8660254037844387076, 1.000000000000000000, 0.8660254037844387076, 1.000000000000000000, 0.8660254037844387076, 1.000000000000000000, 0.8660254037844387076, 1.000000000000000000, 0.8660254037844387076, 1.000000000000000000, 0.8660254037844387076, 1.000000000000000000, 0.8660254037844387076, 1.000000000000000000, 0.9423649185551699059, 0.9343183816103359796),
 ( 1.000000000000000000, 0.8660254037844387076, 1.000000000000000000, 0.8660254037844387076, 1.000000000000000000, 0.8660254037844387076, 1.000000000000000000, 0.8660254037844387076, 1.000000000000000000, 0.8660254037844387076, 1.000000000000000000, 0.8660254037844387076, 1.000000000000000000, 0.8660254037844387076, 1.000000000000000000, 0.8660254037844387076, 1.000000000000000000, 0.8660254037844387076, 1.000000000000000000, 0.8660254037844387076, 1.000000000000000000, 0.8660254037844387076, 1.000000000000000000, 0.8660254037844387076, 1.000000000000000000, 0.8660254037844387076, 1.000000000000000000, 0.8660254037844387076, 1.000000000000000000, 0.8660254037844387076, 1.000000000000000000, 0.8660254037844387076, 1.000000000000000000, 0.8660254037844387076, 1.000000000000000000, 0.8660254037844387076, 1.000000000000000000, 0.8660254037844387076, 1.000000000000000000, 0.8660254037844387076, 1.000000000000000000, 0.8660254037844387076, 1.000000000000000000, 0.8660254037844387076, 1.000000000000000000, 0.8660254037844387076, 1.000000000000000000, 0.8660254037844387076, 1.000000000000000000, 0.8660254037844387076, 1.000000000000000000, 0.8660254037844387076, 1.000000000000000000, 0.8660254037844387076, 1.000000000000000000, 0.8660254037844387076, 1.000000000000000000, 0.8660254037844387076, 1.000000000000000000, 0.8660254037844387076, 1.000000000000000000, 0.8660254037844387076, 1.000000000000000000, 0.8660254037844387076, 1.000000000000000000, 0.8660254037844387076, 1.000000000000000000, 0.8660254037844387076, 1.000000000000000000, 0.8660254037844387076, 1.000000000000000000, 0.8660254037844387076, 1.000000000000000000, 0.8660254037844387076, 1.000000000000000000, 0.8660254037844387076, 1.000000000000000000, 0.8660254037844387076, 1.000000000000000000, 0.8660254037844387076, 1.000000000000000000, 0.8660254037844387076, 1.000000000000000000, 0.8660254037844387076, 1.000000000000000000, 0.8660254037844387076, 1.000000000000000000, 0.8660254037844387076, 1.000000000000000000, 0.8660254037844387076, 1.000000000000000000, 0.8660254037844387076, 1.000000000000000000, 0.8660254037844387076, 1.000000000000000000, 0.8660254037844387076, 1.000000000000000000, 0.8660254037844387076, 1.000000000000000000, 0.8660254037844387076, 1.000000000000000000, 0.8660254037844387076, 1.000000000000000000, 0.9423649185551699059, 0.9343183816103359796) ) ) 
 REPRESENTATION_ITEM ( '' )  SURFACE ( )  );
#9932=CARTESIAN_POINT ( 'NONE',  ( -25.98076211353310683, 53.39374999904394770, -6.871901078670399343 ) ) ;
#9934=CARTESIAN_POINT ( 'NONE',  ( -25.98076211353311393, 49.67499999999986926, -7.309401076758571314 ) ) ;
#9937=CARTESIAN_POINT ( 'NONE',  ( -27.60187600103308014, 55.20208333237728482, -4.064049460664955760 ) ) ;
#9939=ORIENTED_EDGE ( 'NONE', *, *, #553, .F. ) ;
#9943=FACE_OUTER_BOUND ( 'NONE', #9591, .T. ) ;
#9944=ORIENTED_EDGE ( 'NONE', *, *, #5536, .F. ) ;
#9947=( BOUNDED_CURVE ( )  B_SPLINE_CURVE ( 2, ( #7712, #3490, #2717, #4268, #6872, #980, #5162, #4323, #10264 ),
 .UNSPECIFIED., .F., .F. ) 
 B_SPLINE_CURVE_WITH_KNOTS ( ( 3, 2, 2, 2, 3 ),
 ( 0.1944444444444444475, 0.2037037037037036924, 0.2222222222222222099, 0.2407407407407407274, 0.2500000000000000000 ),
 .UNSPECIFIED. ) 
 CURVE ( )  GEOMETRIC_REPRESENTATION_ITEM ( )  RATIONAL_B_SPLINE_CURVE ( ( 0.9330127018922192983, 0.9330127018922194093, 1.000000000000000000, 0.8660254037844387076, 1.000000000000000000, 0.8660254037844387076, 1.000000000000000000, 0.9330127018922191873, 0.9330127018922192983 ) ) 
 REPRESENTATION_ITEM ( '' )  );
#9951=CARTESIAN_POINT ( 'NONE',  ( -24.98076211353312814, 51.62916666475469896, -6.732050807568954909 ) ) ;
#9956=ADVANCED_FACE ( 'NONE', ( #187 ), #2528, .F. ) ;
#9957=EDGE_CURVE ( 'NONE', #101, #2436, #8315, .T. ) ;
#9961=DIRECTION ( 'NONE',  ( 0.000000000000000000, 1.000000000000000000, 0.000000000000000000 ) ) ;
#9962=CYLINDRICAL_SURFACE ( 'NONE', #5537, 1.999999999999971356 ) ;
#9964=CARTESIAN_POINT ( 'NONE',  ( -23.98076211353314235, 51.57083333142138315, -6.154700538379337615 ) ) ;
#9970=CARTESIAN_POINT ( 'NONE',  ( -24.98076211353313170, 52.09583333142136752, -3.267949192431250705 ) ) ;
#9974=CARTESIAN_POINT ( 'NONE',  ( -27.44132332507749439, 55.89336679508493688, -4.296600267573891685 ) ) ;
#9979=VECTOR ( 'NONE', #6932, 1000.000000000000000 ) ;
#9981=CARTESIAN_POINT ( 'NONE',  ( -27.60187600103308725, 50.88541666571061484, -5.935950539335252074 ) ) ;
#9982=CARTESIAN_POINT ( 'NONE',  ( -24.35964822603314772, 52.46041666571062478, -4.064049460664953983 ) ) ;
#9983=EDGE_CURVE ( 'NONE', #2646, #2508, #8818, .T. ) ;
#9985=CARTESIAN_POINT ( 'NONE',  ( -25.98076211353311393, 52.12499999999986500, -2.690598923241634743 ) ) ;
#9997=CARTESIAN_POINT ( 'NONE',  ( -24.35964822603314417, 49.89374999904394770, -5.000000000000103029 ) ) ;
#10000=CARTESIAN_POINT ( 'NONE',  ( -24.98076211353313170, 52.79583333142137036, -3.267949192431250705 ) ) ;
#10009=EDGE_CURVE ( 'NONE', #4732, #6093, #297, .T. ) ;
#10011=CARTESIAN_POINT ( 'NONE',  ( -25.98076211353311393, 50.02499999999987068, -3.000000000000132783 ) ) ;
#10012=CARTESIAN_POINT ( 'NONE',  ( -26.11503144744077076, 56.99999999999888445, -3.000000000000131894 ) ) ;
#10017=AXIS2_PLACEMENT_3D ( 'NONE', #4054, #9097, #1492 ) ;
#10024=CARTESIAN_POINT ( 'NONE',  ( -25.98076211353311393, 53.17499999999985505, -7.000000000000072831 ) ) ;
#10030=FACE_BOUND ( 'NONE', #3672, .T. ) ;
#10031=CARTESIAN_POINT ( 'NONE',  ( -25.98076211353311393, 54.96874999904394343, -6.871901078670400231 ) ) ;
#10032=DIRECTION ( 'NONE',  ( 0.000000000000000000, 1.000000000000000000, 0.000000000000000000 ) ) ;
#10033=CARTESIAN_POINT ( 'NONE',  ( -24.35964822603314417, 49.89374999904394770, -5.000000000000103029 ) ) ;
#10035=ORIENTED_EDGE ( 'NONE', *, *, #6280, .T. ) ;
#10042=CARTESIAN_POINT ( 'NONE',  ( -25.98076211353310683, 54.09374999904395054, -6.871901078670399343 ) ) ;
#10043=AXIS2_PLACEMENT_3D ( 'NONE', #6128, #5252, #2020 ) ;
#10045=CARTESIAN_POINT ( 'NONE',  ( -23.98076211353314235, 52.94166666666653498, -3.845299461620867554 ) ) ;
#10046=ORIENTED_EDGE ( 'NONE', *, *, #8671, .T. ) ;
#10061=CARTESIAN_POINT ( 'NONE',  ( -23.98076211353314235, 54.31249999808803608, -5.000000000000103029 ) ) ;
#10064=PLANE ( 'NONE',  #483 ) ;
#10078=VERTEX_POINT ( 'NONE', #4530 ) ;
#10084=CARTESIAN_POINT ( 'NONE',  ( -27.98076211353308551, 52.00833333333319786, -3.845299461620869330 ) ) ;
#10085=LINE ( 'NONE', #1757, #10939 ) ;
#10090=CARTESIAN_POINT ( 'NONE',  ( -25.98076211353311393, 51.29374999904394627, -6.871901078670400231 ) ) ;
#10100=CARTESIAN_POINT ( 'NONE',  ( -25.98076211353310683, 54.26874999904394059, -6.871901078670399343 ) ) ;
#10101=CARTESIAN_POINT ( 'NONE',  ( -24.35964822603314772, 52.57708333237728482, -5.935950539335252074 ) ) ;
#10102=CARTESIAN_POINT ( 'NONE',  ( -23.98076211353314235, 53.75833333333319786, -6.154700538379337615 ) ) ;
#10105=EDGE_CURVE ( 'NONE', #3014, #3474, #6534, .T. ) ;
#10114=CARTESIAN_POINT ( 'NONE',  ( -25.98076211353311038, 61.49999999999985789, -9.000000000000701661 ) ) ;
#10117=CARTESIAN_POINT ( 'NONE',  ( -24.98076211353312814, 55.12916666475470606, -6.732050807568954909 ) ) ;
#10125=DIRECTION ( 'NONE',  ( 0.000000000000000000, 1.000000000000000000, 0.000000000000000000 ) ) ;
#10126=LINE ( 'NONE', #1512, #9198 ) ;
#10127=LINE ( 'NONE', #2466, #4106 ) ;
#10136=FACE_OUTER_BOUND ( 'NONE', #3739, .T. ) ;
#10137=VECTOR ( 'NONE', #5748, 1000.000000000000000 ) ;
#10142=EDGE_CURVE ( 'NONE', #2370, #8872, #825, .T. ) ;
#10144=CARTESIAN_POINT ( 'NONE',  ( -26.79131905728310059, 55.08541666571061768, -3.596074190997381237 ) ) ;
#10150=FACE_OUTER_BOUND ( 'NONE', #10411, .T. ) ;
#10152=CARTESIAN_POINT ( 'NONE',  ( -25.98076211353310683, 52.51874999904394770, -3.128098921329806714 ) ) ;
#10155=EDGE_CURVE ( 'NONE', #7809, #9774, #9882, .T. ) ;
#10157=CARTESIAN_POINT ( 'NONE',  ( -25.98076211353311393, 53.17499999999985505, -7.309401076758571314 ) ) ;
#10168=CARTESIAN_POINT ( 'NONE',  ( -25.98076211353311393, 55.27499999999985647, -7.000000000000072831 ) ) ;
#10174=CARTESIAN_POINT ( 'NONE',  ( -25.98076211353311393, 54.48749999808803324, -7.309401076758571314 ) ) ;
#10175=ORIENTED_EDGE ( 'NONE', *, *, #9496, .F. ) ;
#10183=CARTESIAN_POINT ( 'NONE',  ( -25.17020516978313083, 52.63541666571061484, -6.403925809002825709 ) ) ;
#10195=CARTESIAN_POINT ( 'NONE',  ( -25.98076211353311393, 52.47499999999985931, -7.000000000000072831 ) ) ;
#10196=CARTESIAN_POINT ( 'NONE',  ( -25.17020516978313083, 51.93541666571061910, -6.403925809002825709 ) ) ;
#10199=FACE_OUTER_BOUND ( 'NONE', #5716, .T. ) ;
#10205=CARTESIAN_POINT ( 'NONE',  ( -24.35964822603314772, 52.75208333237727487, -5.935950539335252074 ) ) ;
#10206=LINE ( 'NONE', #6090, #10728 ) ;
#10209=CARTESIAN_POINT ( 'NONE',  ( -25.98076211353311393, 50.72499999999985931, -2.690598923241634743 ) ) ;
#10216=CARTESIAN_POINT ( 'NONE',  ( -27.44132740410865523, 55.89336612041927310, -4.296608737464627126 ) ) ;
#10219=ORIENTED_EDGE ( 'NONE', *, *, #2230, .T. ) ;
#10222=CIRCLE ( 'NONE', #5959, 1.999999999999971356 ) ;
#10223=EDGE_CURVE ( 'NONE', #6512, #2646, #1945, .T. ) ;
#10224=CARTESIAN_POINT ( 'NONE',  ( -27.98076211353308551, 51.80416666475470322, -6.154700538379338504 ) ) ;
#10225=CARTESIAN_POINT ( 'NONE',  ( -25.17020516978313083, 50.47708333237727629, -3.596074190997380349 ) ) ;
#10228=CARTESIAN_POINT ( 'NONE',  ( -24.35964822603314417, 50.59374999904394343, -5.000000000000103029 ) ) ;
#10232=VERTEX_POINT ( 'NONE', #10791 ) ;
#10236=ORIENTED_EDGE ( 'NONE', *, *, #2878, .F. ) ;
#10242=CARTESIAN_POINT ( 'NONE',  ( -27.60187600103308014, 52.92708333237728624, -4.064049460664955760 ) ) ;
#10255=CARTESIAN_POINT ( 'NONE',  ( -26.79131905728310059, 52.98541666571061626, -3.596074190997381237 ) ) ;
#10262=DIRECTION ( 'NONE',  ( 2.775557561562891351E-17, 1.000000000000000000, -8.326672684688671588E-17 ) ) ;
#10263=CARTESIAN_POINT ( 'NONE',  ( -27.60187600103308725, 52.28541666571061342, -5.935950539335252074 ) ) ;
#10264=CARTESIAN_POINT ( 'NONE',  ( -25.98076211353311393, 51.07499999999986784, -7.000000000000073719 ) ) ;
#10279=CARTESIAN_POINT ( 'NONE',  ( -25.17020516978313083, 52.11041666571060915, -6.403925809002825709 ) ) ;
#10284=EDGE_CURVE ( 'NONE', #6644, #3608, #509, .T. ) ;
#10285=CARTESIAN_POINT ( 'NONE',  ( -27.98076211353308551, 54.02083333142136468, -3.845299461620869330 ) ) ;
#10297=CARTESIAN_POINT ( 'NONE',  ( -25.17020516978313083, 51.00208333237728198, -3.596074190997380349 ) ) ;
#10310=CARTESIAN_POINT ( 'NONE',  ( -26.79131905728310059, 54.85208333237729050, -6.403925809002825709 ) ) ;
#10312=CARTESIAN_POINT ( 'NONE',  ( -25.18193375740463935, 57.38490676151830172, -3.163901733045028752 ) ) ;
#10316=AXIS2_PLACEMENT_3D ( 'NONE', #2530, #5862, #8302 ) ;
#10320=CARTESIAN_POINT ( 'NONE',  ( -24.35964822603314772, 54.85208333237728340, -5.935950539335252074 ) ) ;
#10327=CARTESIAN_POINT ( 'NONE',  ( -26.51666049839534622, 54.89373926088290290, -3.000000000000131006 ) ) ;
#10336=CARTESIAN_POINT ( 'NONE',  ( -25.98076211353311393, 51.46874999904394343, -6.871901078670400231 ) ) ;
#10348=CARTESIAN_POINT ( 'NONE',  ( -26.79131905728310059, 49.95208333237728482, -6.403925809002825709 ) ) ;
#10351=CARTESIAN_POINT ( 'NONE',  ( -26.92841756856055824, 58.32602275755382948, -6.761469286193118933 ) ) ;
#10352=ORIENTED_EDGE ( 'NONE', *, *, #4025, .F. ) ;
#10357=DIRECTION ( 'NONE',  ( 0.000000000000000000, 0.000000000000000000, 1.000000000000000000 ) ) ;
#10358=( BOUNDED_CURVE ( )  B_SPLINE_CURVE ( 2, ( #5084, #4075, #3298, #8346, #5851, #9964, #6736, #9233, #5028 ),
 .UNSPECIFIED., .F., .F. ) 
 B_SPLINE_CURVE_WITH_KNOTS ( ( 3, 2, 2, 2, 3 ),
 ( 0.1944444444444444198, 0.2037037037037036924, 0.2222222222222222099, 0.2407407407407407274, 0.2500000000000000000 ),
 .UNSPECIFIED. ) 
 CURVE ( )  GEOMETRIC_REPRESENTATION_ITEM ( )  RATIONAL_B_SPLINE_CURVE ( ( 0.9330127018922192983, 0.9330127018922191873, 1.000000000000000000, 0.8660254037844387076, 1.000000000000000000, 0.8660254037844387076, 1.000000000000000000, 0.9330127018922191873, 0.9330127018922192983 ) ) 
 REPRESENTATION_ITEM ( '' )  );
#10362=CARTESIAN_POINT ( 'NONE',  ( -27.60187600103308370, 52.16874999904395338, -5.000000000000103029 ) ) ;
#10365=AXIS2_PLACEMENT_3D ( 'NONE', #7152, #5499, #5382 ) ;
#10370=CARTESIAN_POINT ( 'NONE',  ( -25.98076211353311749, 56.99999999999884182, -7.000000000000094147 ) ) ;
#10371=CARTESIAN_POINT ( 'NONE',  ( -25.44486372867087809, 55.24373926088289721, -7.000000000000075495 ) ) ;
#10375=ORIENTED_EDGE ( 'NONE', *, *, #8639, .F. ) ;
#10377=ORIENTED_EDGE ( 'NONE', *, *, #293, .T. ) ;
#10382=EDGE_CURVE ( 'NONE', #5854, #6011, #1741, .T. ) ;
#10390=DIRECTION ( 'NONE',  ( 1.000000000000000000, 0.000000000000000000, -0.000000000000000000 ) ) ;
#10391=CARTESIAN_POINT ( 'NONE',  ( -25.17020516978313083, 51.41041666571061342, -6.403925809002825709 ) ) ;
#10405=CARTESIAN_POINT ( 'NONE',  ( -24.35964822603314417, 51.11874999904394912, -5.000000000000103029 ) ) ;
#10411=EDGE_LOOP ( 'NONE', ( #3157, #5170, #67, #2749 ) ) ;
#10413=CYLINDRICAL_SURFACE ( 'NONE', #10043, 1.999999999999971356 ) ;
#10417=CARTESIAN_POINT ( 'NONE',  ( -26.98076211353408382, 57.99999999999985789, -3.267949192431818251 ) ) ;
#10424=CARTESIAN_POINT ( 'NONE',  ( -26.98076211353408382, 57.99999999999985789, -3.267949192431818251 ) ) ;
#10428=( BOUNDED_CURVE ( )  B_SPLINE_CURVE ( 2, ( #2075, #7176, #6233, #1121, #8854 ),
 .UNSPECIFIED., .F., .F. ) 
 B_SPLINE_CURVE_WITH_KNOTS ( ( 3, 2, 3 ),
 ( 0.000000000000000000, 0.01851851851851851749, 0.02777777777777777971 ),
 .UNSPECIFIED. ) 
 CURVE ( )  GEOMETRIC_REPRESENTATION_ITEM ( )  RATIONAL_B_SPLINE_CURVE ( ( 1.000000000000000000, 0.8660254037844387076, 1.000000000000000000, 0.9330127018922192983, 0.9330127018922194093 ) ) 
 REPRESENTATION_ITEM ( '' )  );
#10440=VERTEX_POINT ( 'NONE', #4244 ) ;
#10441=EDGE_LOOP ( 'NONE', ( #770, #1241, #10659, #1192, #1306, #2471 ) ) ;
#10443=EDGE_CURVE ( 'NONE', #2547, #2239, #9196, .T. ) ;
#10454=CARTESIAN_POINT ( 'NONE',  ( -25.17020516978313083, 52.57708333237728482, -3.596074190997380349 ) ) ;
#10460=ORIENTED_EDGE ( 'NONE', *, *, #6280, .F. ) ;
#10465=CARTESIAN_POINT ( 'NONE',  ( -25.17020516978313083, 55.20208333237728482, -3.596074190997380349 ) ) ;
#10469=ORIENTED_EDGE ( 'NONE', *, *, #10803, .F. ) ;
#10478=SURFACE_STYLE_USAGE ( .BOTH. , #243 ) ;
#10488=CARTESIAN_POINT ( 'NONE',  ( -23.98076211353314235, 53.05833333333319501, -6.154700538379337615 ) ) ;
#10490=CARTESIAN_POINT ( 'NONE',  ( -26.98076211353309972, 51.36666666666653214, -3.267949192431252037 ) ) ;
#10491=CARTESIAN_POINT ( 'NONE',  ( -26.79131905728310059, 54.32708333237727771, -6.403925809002825709 ) ) ;
#10492=B_SPLINE_CURVE_WITH_KNOTS ( 'NONE', 3,
 ( #6032, #6750, #2533, #5208, #5918, #10312, #2708, #6083, #9472, #8644 ),
 .UNSPECIFIED., .F., .F.,
 ( 4, 2, 2, 2, 4 ),
 ( 6.952433221959954168E-18, 0.0003978633013915846856, 0.0007957266027831624323, 0.001193589904174740179, 0.001591453205566317926 ),
 .UNSPECIFIED. ) ;
#10494=CARTESIAN_POINT ( 'NONE',  ( -23.98076211353314235, 55.15833333333319644, -6.154700538379337615 ) ) ;
#10497=CARTESIAN_POINT ( 'NONE',  ( -25.98076211353311393, 50.63749999808803892, -3.000000000000132339 ) ) ;
#10504=VECTOR ( 'NONE', #2244, 1000.000000000000000 ) ;
#10505=CARTESIAN_POINT ( 'NONE',  ( -24.35964822603314772, 50.36041666571061626, -4.064049460664953983 ) ) ;
#10508=CARTESIAN_POINT ( 'NONE',  ( -25.17020516978313083, 54.21041666571061057, -6.403925809002825709 ) ) ;
#10517=CARTESIAN_POINT ( 'NONE',  ( -27.44132332588852918, 55.71836679495081057, -4.296600269257925930 ) ) ;
#10529=CARTESIAN_POINT ( 'NONE',  ( -27.44132740410865523, 55.89336612041927310, -4.296608737464627126 ) ) ;
#10530=CARTESIAN_POINT ( 'NONE',  ( -27.60187600103308014, 55.69181177618367684, -4.629976867109323990 ) ) ;
#10533=CYLINDRICAL_SURFACE ( 'NONE', #8441, 1.999999999999971356 ) ;
#10542=CARTESIAN_POINT ( 'NONE',  ( -27.60187600103308370, 52.34374999904394343, -5.000000000000103029 ) ) ;
#10544=CARTESIAN_POINT ( 'NONE',  ( -27.98076211353308551, 55.39166666666653072, -6.154700538379338504 ) ) ;
#10546=CARTESIAN_POINT ( 'NONE',  ( -26.51666049839535688, 54.60626073911682710, -7.000000000000071942 ) ) ;
#10548=ORIENTED_EDGE ( 'NONE', *, *, #2819, .F. ) ;
#10549=AXIS2_PLACEMENT_3D ( 'NONE', #2375, #8268, #651 ) ;
#10550=LINE ( 'NONE', #9599, #1877 ) ;
#10558=CARTESIAN_POINT ( 'NONE',  ( -24.35964822603314417, 54.79374999904394627, -5.000000000000103029 ) ) ;
#10583=CARTESIAN_POINT ( 'NONE',  ( -26.77998953358746803, 58.61463389606510788, -3.164065525718655181 ) ) ;
#10584=CARTESIAN_POINT ( 'NONE',  ( -26.98076211353309972, 49.73333333333319928, -6.732050807568954909 ) ) ;
#10598=CARTESIAN_POINT ( 'NONE',  ( -27.60187600103308014, 52.28541666571061342, -5.935950539335252074 ) ) ;
#10601=ORIENTED_EDGE ( 'NONE', *, *, #10284, .T. ) ;
#10607=CARTESIAN_POINT ( 'NONE',  ( -25.98076211353310683, 50.59374999904395054, -6.871901078670399343 ) ) ;
#10610=EDGE_CURVE ( 'NONE', #8872, #998, #4213, .T. ) ;
#10621=STYLED_ITEM ( 'NONE', ( #7818 ), #1846 ) ;
#10628=CARTESIAN_POINT ( 'NONE',  ( -26.98076211353309972, 52.67916666475470322, -3.267949192431252037 ) ) ;
#10639=CARTESIAN_POINT ( 'NONE',  ( -25.36430081112252211, 57.20223309010732748, -6.905092627761828972 ) ) ;
#10651=CARTESIAN_POINT ( 'NONE',  ( -26.98076211353309972, 51.13333333333319786, -6.732050807568954909 ) ) ;
#10652=CARTESIAN_POINT ( 'NONE',  ( -25.98076211353311393, 50.76874999904394770, -6.871901078670400231 ) ) ;
#10656=CARTESIAN_POINT ( 'NONE',  ( -24.98076211353313170, 54.19583333142136894, -3.267949192431250705 ) ) ;
#10659=ORIENTED_EDGE ( 'NONE', *, *, #10443, .T. ) ;
#10675=CARTESIAN_POINT ( 'NONE',  ( -23.98076211353314235, 52.97083333142136041, -6.154700538379337615 ) ) ;
#10684=CARTESIAN_POINT ( 'NONE',  ( -27.98076211353308551, 52.56249999808803608, -5.000000000000103029 ) ) ;
#10695=DIRECTION ( 'NONE',  ( 0.000000000000000000, 1.000000000000000000, 0.000000000000000000 ) ) ;
#10698=CARTESIAN_POINT ( 'NONE',  ( -25.98076211353311393, 50.94374999904395196, -3.128098921329806714 ) ) ;
#10704=CARTESIAN_POINT ( 'NONE',  ( -24.35964822603314772, 50.65208333237728056, -5.935950539335252074 ) ) ;
#10705=CARTESIAN_POINT ( 'NONE',  ( -27.60187600103308725, 54.32708333237728482, -4.064049460664955760 ) ) ;
#10707=CARTESIAN_POINT ( 'NONE',  ( -27.60187600103308014, 55.02708333237728056, -4.064049460664955760 ) ) ;
#10712=ORIENTED_EDGE ( 'NONE', *, *, #1537, .T. ) ;
#10713=CARTESIAN_POINT ( 'NONE',  ( -25.98076211353311393, 49.49999999999986500, -5.000000000000103029 ) ) ;
#10720=CARTESIAN_POINT ( 'NONE',  ( -27.98076211353308551, 53.32083333142136894, -3.845299461620869330 ) ) ;
#10722=CARTESIAN_POINT ( 'NONE',  ( -26.98076211353309972, 53.46666666666653356, -3.267949192431252037 ) ) ;
#10728=VECTOR ( 'NONE', #3548, 1000.000000000000000 ) ;
#10729=CARTESIAN_POINT ( 'NONE',  ( -24.98076211353313170, 52.18333333333320212, -3.267949192431250705 ) ) ;
#10733=CARTESIAN_POINT ( 'NONE',  ( -26.59698951503823139, 57.20194332867976073, -3.094806908524387445 ) ) ;
#10743=CYLINDRICAL_SURFACE ( 'NONE', #1904, 1.999999999999971356 ) ;
#10744=CARTESIAN_POINT ( 'NONE',  ( -25.44486372867087098, 52.06876073720499676, -3.000000000000133227 ) ) ;
#10748=CARTESIAN_POINT ( 'NONE',  ( -24.35964822603314772, 49.77708333237728766, -5.935950539335252074 ) ) ;
#10749=EDGE_CURVE ( 'NONE', #5575, #1944, #5887, .T. ) ;
#10750=DIRECTION ( 'NONE',  ( 0.000000000000000000, 1.000000000000000000, 0.000000000000000000 ) ) ;
#10756=DIRECTION ( 'NONE',  ( 0.000000000000000000, 0.000000000000000000, 1.000000000000000000 ) ) ;
#10757=CARTESIAN_POINT ( 'NONE',  ( -25.98076211353310683, 50.76874999904394770, -6.871901078670399343 ) ) ;
#10759=CARTESIAN_POINT ( 'NONE',  ( -24.35964822603314772, 53.27708333237728056, -5.935950539335252074 ) ) ;
#10762=CARTESIAN_POINT ( 'NONE',  ( -24.35964822603314772, 54.56041666571061910, -4.064049460664953983 ) ) ;
#10768=ORIENTED_EDGE ( 'NONE', *, *, #2908, .F. ) ;
#10780=CARTESIAN_POINT ( 'NONE',  ( -23.98076211353314235, 51.51249999808803182, -5.000000000000103029 ) ) ;
#10788=B_SPLINE_CURVE_WITH_KNOTS ( 'NONE', 3,
 ( #3579, #9353, #1749, #4303, #10351, #65, #6852, #1803, #6125, #2862, #2180, #1239 ),
 .UNSPECIFIED., .F., .F.,
 ( 4, 2, 2, 2, 2, 4 ),
 ( 0.003180596909393765097, 0.003379140308194210698, 0.003577683706994655866, 0.003974770504595546636, 0.004371857302196437839, 0.004768944099797328175 ),
 .UNSPECIFIED. ) ;
#10791=CARTESIAN_POINT ( 'NONE',  ( -25.98076211353311393, 51.07499999999986784, -7.000000000000073719 ) ) ;
#10794=DIRECTION ( 'NONE',  ( 0.000000000000000000, 1.000000000000000000, 0.000000000000000000 ) ) ;
#10803=EDGE_CURVE ( 'NONE', #998, #5599, #5835, .T. ) ;
#10807=CARTESIAN_POINT ( 'NONE',  ( -25.98076211353311393, 54.61874999904394912, -3.128098921329806714 ) ) ;
#10815=LINE ( 'NONE', #6477, #2216 ) ;
#10816=CARTESIAN_POINT ( 'NONE',  ( -27.60187600103308725, 52.22708333237728340, -4.064049460664955760 ) ) ;
#10818=CARTESIAN_POINT ( 'NONE',  ( -25.98076211353311393, 51.42499999999986215, -2.690598923241634743 ) ) ;
#10826=EDGE_CURVE ( 'NONE', #9873, #1738, #8386, .T. ) ;
#10836=CARTESIAN_POINT ( 'NONE',  ( -26.98076211353309972, 51.74583333142136610, -6.732050807568954909 ) ) ;
#10838=CARTESIAN_POINT ( 'NONE',  ( -26.51666049839535688, 51.30623925897106830, -3.000000000000134115 ) ) ;
#10850=CARTESIAN_POINT ( 'NONE',  ( -27.98076211353308551, 55.36249999808803324, -5.000000000000103029 ) ) ;
#10853=ADVANCED_FACE ( 'NONE', ( #4282 ), #4573, .T. ) ;
#10858=CARTESIAN_POINT ( 'NONE',  ( -25.98076211353311038, 61.49999999999985789, -5.000000000000102141 ) ) ;
#10860=CARTESIAN_POINT ( 'NONE',  ( -25.17020516978313083, 55.61041666571061626, -6.403925809002825709 ) ) ;
#10868=CARTESIAN_POINT ( 'NONE',  ( -27.60187600103308725, 51.58541666571061057, -5.935950539335252074 ) ) ;
#10869=CARTESIAN_POINT ( 'NONE',  ( -24.35964822603314772, 53.86041666571061626, -4.064049460664953983 ) ) ;
#10871=CARTESIAN_POINT ( 'NONE',  ( -24.98076211353313170, 52.88333333333319786, -3.267949192431250705 ) ) ;
#10877=VERTEX_POINT ( 'NONE', #2923 ) ;
#10879=VERTEX_POINT ( 'NONE', #4485 ) ;
#10883=CARTESIAN_POINT ( 'NONE',  ( -27.60187600103308014, 50.18541666571061199, -5.935950539335252074 ) ) ;
#10887=CARTESIAN_POINT ( 'NONE',  ( -25.98076211353311393, 50.41874999904393917, -3.128098921329806714 ) ) ;
#10889=ORIENTED_EDGE ( 'NONE', *, *, #4850, .F. ) ;
#10894=ORIENTED_EDGE ( 'NONE', *, *, #409, .F. ) ;
#10898=CARTESIAN_POINT ( 'NONE',  ( -24.98076211353213694, 57.99999999999985789, -6.732050807568384698 ) ) ;
#10903=AXIS2_PLACEMENT_3D ( 'NONE', #2945, #6260, #1214 ) ;
#10909=DIRECTION ( 'NONE',  ( 0.000000000000000000, 0.000000000000000000, 1.000000000000000000 ) ) ;
#10910=CARTESIAN_POINT ( 'NONE',  ( -25.98076211353311393, 54.48749999808803324, -7.000000000000072831 ) ) ;
#10917=CARTESIAN_POINT ( 'NONE',  ( -24.35964822603314772, 51.17708333237728624, -5.935950539335252074 ) ) ;
#10923=DIRECTION ( 'NONE',  ( 0.000000000000000000, 0.000000000000000000, -1.000000000000000000 ) ) ;
#10924=CARTESIAN_POINT ( 'NONE',  ( -26.51666049839535688, 53.90626073911682425, -7.000000000000071942 ) ) ;
#10925=CARTESIAN_POINT ( 'NONE',  ( -27.60187600103308725, 53.80208333237728624, -4.064049460664955760 ) ) ;
#10926=CARTESIAN_POINT ( 'NONE',  ( -25.17020516978313083, 54.73541666571062336, -6.403925809002825709 ) ) ;
#10929=CARTESIAN_POINT ( 'NONE',  ( -27.98076211353308551, 52.00833333333319786, -3.845299461620869330 ) ) ;
#10939=VECTOR ( 'NONE', #8408, 1000.000000000000000 ) ;
#10946=CARTESIAN_POINT ( 'NONE',  ( -26.98076211353309972, 54.77916666475469754, -3.267949192431252037 ) ) ;
#10950=ORIENTED_EDGE ( 'NONE', *, *, #8581, .T. ) ;
#10962=CARTESIAN_POINT ( 'NONE',  ( -25.98076211353311749, 56.99999999999886313, -3.000000000000122569 ) ) ;
#10979=CARTESIAN_POINT ( 'NONE',  ( -25.17020516978313083, 53.33541666571061768, -6.403925809002825709 ) ) ;
#10984=CARTESIAN_POINT ( 'NONE',  ( -26.98076211353309972, 50.66666666666652930, -3.267949192431252037 ) ) ;
#10986=CARTESIAN_POINT ( 'NONE',  ( -27.60187600103308725, 54.50208333237726777, -4.064049460664955760 ) ) ;
#10987=CARTESIAN_POINT ( 'NONE',  ( -26.79131905728310059, 55.55208333237728624, -6.403925809002825709 ) ) ;
#10989=CARTESIAN_POINT ( 'NONE',  ( -26.98076211353309972, 51.36666666666653214, -3.267949192431252037 ) ) ;
#10991=ORIENTED_EDGE ( 'NONE', *, *, #7977, .F. ) ;
#10992=VERTEX_POINT ( 'NONE', #2818 ) ;
#10995=ORIENTED_EDGE ( 'NONE', *, *, #7443, .F. ) ;
ENDSEC;
END-ISO-10303-21;
